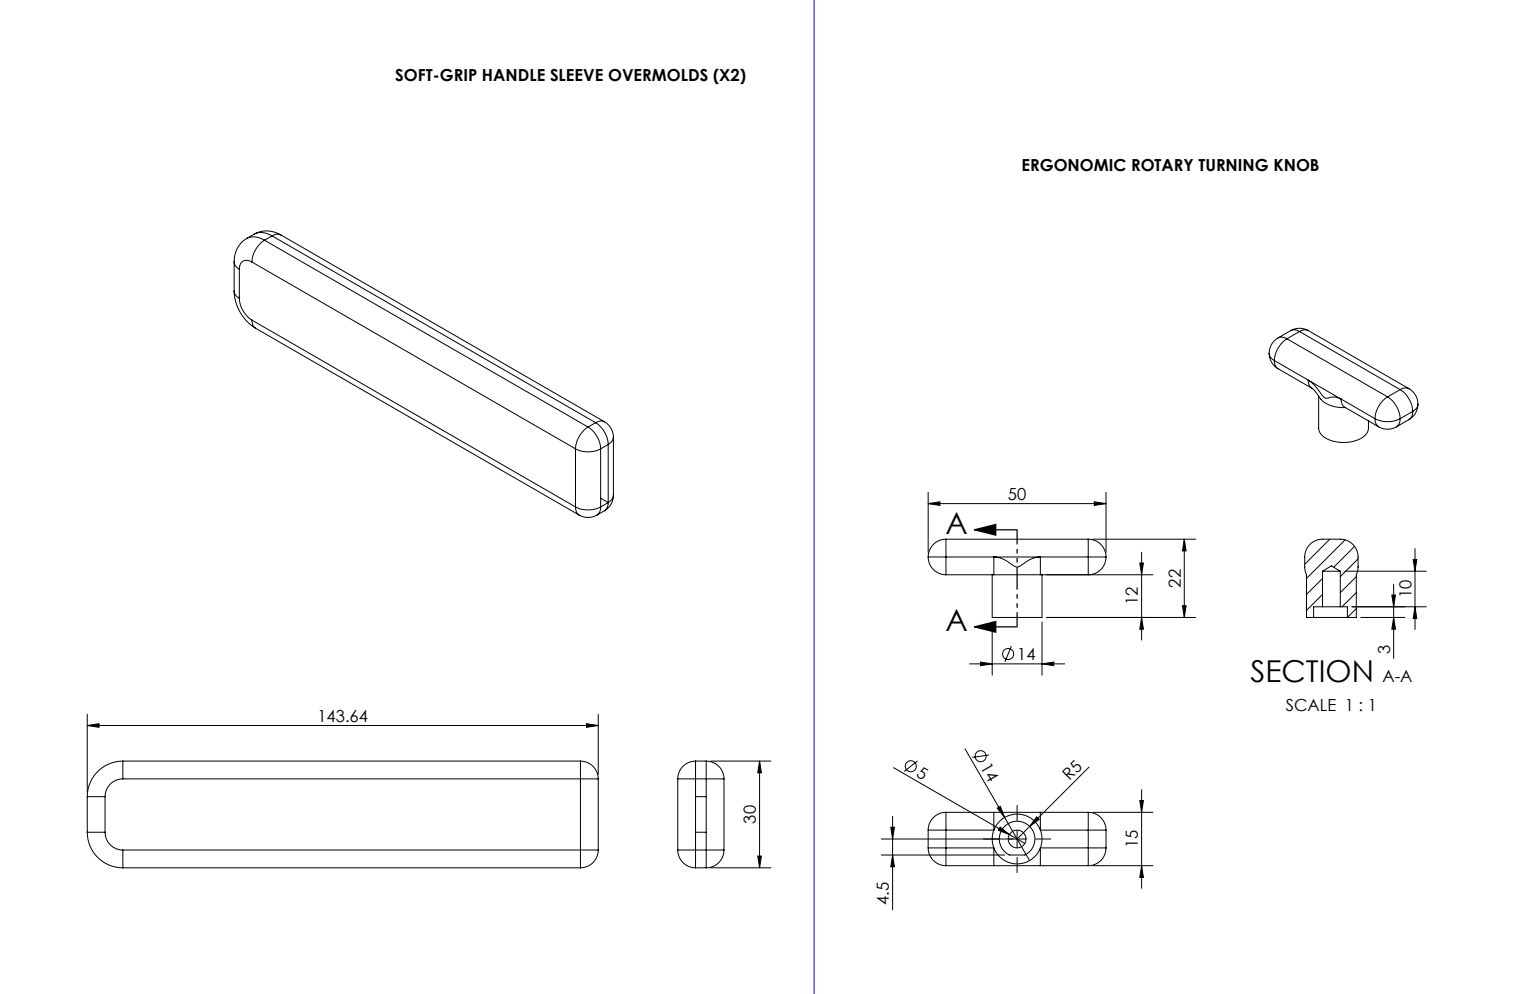
ISO-10303-21;
HEADER;
FILE_DESCRIPTION (('STEP AP214'),
    '1' );
FILE_NAME ('Ergonomic Rotary Turning Knob.step',
    '2026-09-24T10:15:42',
    ( '' ),
    ( '' ),
    'SwSTEP 2.0',
    'SolidWorks 2026',
    '' );
FILE_SCHEMA (( 'AUTOMOTIVE_DESIGN' ));
ENDSEC;

DATA;
#13=CARTESIAN_POINT ( 'NONE',  ( 6.538348415311012296, -7.500000000000000888, -12.00000000000000000 ) ) ;
#17=DIRECTION ( 'NONE',  ( 1.000000000000000000, 0.000000000000000000, 0.000000000000000000 ) ) ;
#23=( BOUNDED_SURFACE ( )  B_SPLINE_SURFACE ( 3, 2, ( 
 ( #9096, #13, #15967 ),
 ( #13391, #10337, #14824 ),
 ( #11773, #4513, #14919 ),
 ( #3147, #1737, #16166 ),
 ( #3050, #14723, #10241 ),
 ( #5830, #6041, #1634 ),
 ( #16367, #7585, #7479 ),
 ( #8709, #13293, #11868 ),
 ( #17403, #308, #4405 ),
 ( #11673, #17708, #11585 ),
 ( #4605, #13483, #14634 ),
 ( #10432, #2857, #16066 ),
 ( #10529, #6137, #4319 ),
 ( #1837, #2958, #14535 ),
 ( #11963, #3250, #7675 ),
 ( #1450, #8805, #1543 ),
 ( #7383, #112, #18081 ),
 ( #4980, #16642, #4896 ),
 ( #1935, #13772, #10817 ),
 ( #3545, #6425, #502 ),
 ( #15014, #6332, #12161 ),
 ( #13684, #7870, #13859 ),
 ( #12251, #7768, #685 ),
 ( #777, #6517, #13581 ),
 ( #598, #3730, #9385 ),
 ( #16464, #9186, #5164 ),
 ( #6228, #10723, #12335 ),
 ( #2209, #3349, #8051 ),
 ( #15212, #12061, #18171 ),
 ( #17895, #2122, #17990 ),
 ( #7963, #5070, #3447 ),
 ( #15113, #9558, #10920 ),
 ( #16558, #16740, #4798 ),
 ( #3639, #11009, #16826 ),
 ( #9474, #15389, #9281 ),
 ( #15296, #6610, #2295 ),
 ( #12433, #18262, #8141 ),
 ( #399, #10633, #2029 ),
 ( #867, #11100, #16916 ),
 ( #5524, #4007, #17020 ),
 ( #5350, #5441, #11374 ),
 ( #2657, #12703, #11287 ),
 ( #17193, #15481, #8406 ),
 ( #6984, #18535, #1038 ) ),
 .UNSPECIFIED., .F., .F., .T. ) 
 B_SPLINE_SURFACE_WITH_KNOTS ( ( 4, 2, 2, 2, 2, 2, 2, 2, 2, 2, 2, 2, 2, 2, 2, 2, 2, 2, 2, 2, 2, 4 ),
 ( 3, 3 ),
 ( 0.007984881688765531685, 0.008880023643941203221, 0.009775165599116873022, 0.01067030755429254282, 0.01156544950946821262, 0.01246059146464388243, 0.01335573341981955396, 0.01425087537499522550, 0.01469844635258306040, 0.01492223184137697785, 0.01514601733017089530, 0.01536980281896481275, 0.01559358830775873020, 0.01581737379655264591, 0.01604115928534656510, 0.01693630124052223490, 0.01783144319569790470, 0.01872658515087357797, 0.01962172710604925124, 0.02051686906122492104, 0.02141201101640059085, 0.02230715297157626065 ),
 ( 0.000000000000000000, 1.000000000000000000 ),
 .UNSPECIFIED. ) 
 GEOMETRIC_REPRESENTATION_ITEM ( )  RATIONAL_B_SPLINE_SURFACE ( (
 ( 1.000000000000000000, 0.7071067811865474617, 1.000000000000000000),
 ( 1.000000000000000000, 0.7141735847353027911, 1.000000000000000000),
 ( 1.000000000000000000, 0.7220150969518837059, 1.000000000000000000),
 ( 1.000000000000000000, 0.7390483610380735868, 1.000000000000000000),
 ( 1.000000000000000000, 0.7482852340371979327, 1.000000000000000000),
 ( 1.000000000000000000, 0.7685052920442676516, 1.000000000000000000),
 ( 1.000000000000000000, 0.7795547470752138830, 1.000000000000000000),
 ( 1.000000000000000000, 0.8031735375541008137, 1.000000000000000000),
 ( 1.000000000000000000, 0.8157770400072400507, 1.000000000000000000),
 ( 1.000000000000000000, 0.8424364036431882807, 1.000000000000000000),
 ( 1.000000000000000000, 0.8565278543580017168, 1.000000000000000000),
 ( 1.000000000000000000, 0.8853337094945018526, 1.000000000000000000),
 ( 1.000000000000000000, 0.9000757013528668526, 1.000000000000000000),
 ( 1.000000000000000000, 0.9285356150544983311, 1.000000000000000000),
 ( 1.000000000000000000, 0.9423225300521810288, 1.000000000000000000),
 ( 1.000000000000000000, 0.9592421851076473605, 1.000000000000000000),
 ( 1.000000000000000000, 0.9642414584271679079, 1.000000000000000000),
 ( 1.000000000000000000, 0.9699277023943830844, 1.000000000000000000),
 ( 1.000000000000000000, 0.9715166551480127755, 1.000000000000000000),
 ( 1.000000000000000000, 0.9737696706145027026, 1.000000000000000000),
 ( 1.000000000000000000, 0.9744508395083844032, 1.000000000000000000),
 ( 1.000000000000000000, 0.9748110790397115366, 1.000000000000000000),
 ( 1.000000000000000000, 0.9744748476087098377, 1.000000000000000000),
 ( 1.000000000000000000, 0.9728601655991807595, 1.000000000000000000),
 ( 1.000000000000000000, 0.9715893508620213614, 1.000000000000000000),
 ( 1.000000000000000000, 0.9682746065025299442, 1.000000000000000000),
 ( 1.000000000000000000, 0.9662330922797159882, 1.000000000000000000),
 ( 1.000000000000000000, 0.9616633680012534047, 1.000000000000000000),
 ( 1.000000000000000000, 0.9591230388079813318, 1.000000000000000000),
 ( 1.000000000000000000, 0.9454866025348970249, 1.000000000000000000),
 ( 1.000000000000000000, 0.9317605398179185094, 1.000000000000000000),
 ( 1.000000000000000000, 0.9032287473899394126, 1.000000000000000000),
 ( 1.000000000000000000, 0.8883390392773794497, 1.000000000000000000),
 ( 1.000000000000000000, 0.8592388025803222584, 1.000000000000000000),
 ( 1.000000000000000000, 0.8450030273492604715, 1.000000000000000000),
 ( 1.000000000000000000, 0.8179255325836626289, 1.000000000000000000),
 ( 1.000000000000000000, 0.8050698650503591569, 1.000000000000000000),
 ( 1.000000000000000000, 0.7808988731588855092, 1.000000000000000000),
 ( 1.000000000000000000, 0.7696290231168715357, 1.000000000000000000),
 ( 1.000000000000000000, 0.7490294503509588031, 1.000000000000000000),
 ( 1.000000000000000000, 0.7396188834547082758, 1.000000000000000000),
 ( 1.000000000000000000, 0.7222670797466549386, 1.000000000000000000),
 ( 1.000000000000000000, 0.7142721232192638103, 1.000000000000000000),
 ( 1.000000000000000000, 0.7071067811865517916, 1.000000000000000000) ) ) 
 REPRESENTATION_ITEM ( '' )  SURFACE ( )  );
#91=B_SPLINE_CURVE_WITH_KNOTS ( 'NONE', 3,
 ( #3030, #15094, #17687, #2012, #6309, #12042, #7847, #10410, #3227, #4588, #16446, #8878, #7562, #11849, #12235, #14704, #7462, #16246, #1615, #18061, #4965, #7658, #8974, #13373, #10511, #16347, #7751, #17876, #9076, #3330, #14902, #9169, #1913, #12143, #13561, #12586, #2450, #12411 ),
 .UNSPECIFIED., .F., .F.,
 ( 4, 2, 2, 2, 2, 2, 2, 2, 2, 2, 2, 2, 2, 2, 2, 2, 2, 2, 4 ),
 ( 0.000000000000000000, 0.0009058109605214417380, 0.001811621921042883476, 0.002717432881564325105, 0.003623243842085765217, 0.004529054802607205762, 0.005434865763128644139, 0.006340676723650081649, 0.006793582203910802572, 0.007246487684171522628, 0.007699393164432242684, 0.008152298644692964474, 0.009058109605214402851, 0.009963920565735844698, 0.01086973152625728828, 0.01177554248677873013, 0.01268135344730017371, 0.01358716440782161729, 0.01449297536834306087 ),
 .UNSPECIFIED. ) ;
#94=CARTESIAN_POINT ( 'NONE',  ( 0.000000000000000000, 0.000000000000000000, -3.000000000000000000 ) ) ;
#97=CARTESIAN_POINT ( 'NONE',  ( -6.538348415311006967, 7.499999999999999112, -17.00000000000000000 ) ) ;
#100=CARTESIAN_POINT ( 'NONE',  ( -6.538348415310934136, -2.500000000000000444, -17.00000000000101252 ) ) ;
#105=EDGE_LOOP ( 'NONE', ( #11918, #3838, #18012, #4953 ) ) ;
#112=CARTESIAN_POINT ( 'NONE',  ( 1.213280723413316275, -7.500000000000199840, -13.07603167631435603 ) ) ;
#115=DIRECTION ( 'NONE',  ( 0.000000000000000000, 0.000000000000000000, 1.000000000000000000 ) ) ;
#128=ORIENTED_EDGE ( 'NONE', *, *, #3767, .F. ) ;
#158=ORIENTED_EDGE ( 'NONE', *, *, #3779, .F. ) ;
#183=ORIENTED_EDGE ( 'NONE', *, *, #15931, .F. ) ;
#186=DIRECTION ( 'NONE',  ( 0.000000000000000000, 0.000000000000000000, -1.000000000000000000 ) ) ;
#189=DIRECTION ( 'NONE',  ( -1.000000000000000000, -8.673617379884033500E-16, 0.000000000000000000 ) ) ;
#194=CARTESIAN_POINT ( 'NONE',  ( 25.00000000000000000, 7.499999999999999112, -16.99999999999999645 ) ) ;
#197=ORIENTED_EDGE ( 'NONE', *, *, #8046, .T. ) ;
#226=AXIS2_PLACEMENT_3D ( 'NONE', #9917, #9039, #13430 ) ;
#229=CARTESIAN_POINT ( 'NONE',  ( 0.000000000000000000, 0.000000000000000000, -12.00000000000000000 ) ) ;
#230=EDGE_LOOP ( 'NONE', ( #7603, #4176, #7702, #11957 ) ) ;
#232=ORIENTED_EDGE ( 'NONE', *, *, #17218, .F. ) ;
#253=ORIENTED_EDGE ( 'NONE', *, *, #15488, .F. ) ;
#270=CARTESIAN_POINT ( 'NONE',  ( 2.179449471770337432, -4.500000000000000000, -3.000000000000000000 ) ) ;
#289=DIRECTION ( 'NONE',  ( -0.000000000000000000, -0.000000000000000000, 1.000000000000000000 ) ) ;
#290=CARTESIAN_POINT ( 'NONE',  ( -5.935721797379079234, 7.499999999999999112, -16.97606798286715701 ) ) ;
#298=AXIS2_PLACEMENT_3D ( 'NONE', #7660, #11852, #11947 ) ;
#308=CARTESIAN_POINT ( 'NONE',  ( 5.084818453916919445, -7.499999999999999112, -13.03762002034291534 ) ) ;
#316=DIRECTION ( 'NONE',  ( -1.000000000000000000, 1.734723475976806848E-16, 0.000000000000000000 ) ) ;
#322=VERTEX_POINT ( 'NONE', #3941 ) ;
#370=ORIENTED_EDGE ( 'NONE', *, *, #6465, .T. ) ;
#376=DIRECTION ( 'NONE',  ( 0.000000000000000000, -0.000000000000000000, 1.000000000000000000 ) ) ;
#393=ORIENTED_EDGE ( 'NONE', *, *, #1315, .T. ) ;
#394=CARTESIAN_POINT ( 'NONE',  ( 20.00000000000000000, -2.500000000000000444, -17.00000000000000000 ) ) ;
#399=CARTESIAN_POINT ( 'NONE',  ( -6.009712068683241704, -3.596569907853852666, -12.00000000129638345 ) ) ;
#412=DIRECTION ( 'NONE',  ( 1.000000000000000000, -0.000000000000000000, -0.000000000000000000 ) ) ;
#435=SURFACE_STYLE_USAGE ( .BOTH. , #6368 ) ;
#437=DIRECTION ( 'NONE',  ( -0.000000000000000000, -1.000000000000000000, -0.000000000000000000 ) ) ;
#465=DIRECTION ( 'NONE',  ( -1.000000000000000000, -0.000000000000000000, -0.000000000000000000 ) ) ;
#467=DIRECTION ( 'NONE',  ( 1.000000000000000000, 0.000000000000000000, -0.000000000000000000 ) ) ;
#481=ORIENTED_EDGE ( 'NONE', *, *, #8485, .T. ) ;
#483=FACE_OUTER_BOUND ( 'NONE', #969, .T. ) ;
#502=CARTESIAN_POINT ( 'NONE',  ( 0.1927609796801927344, -7.500000000000000888, -14.19253746125320781 ) ) ;
#528=AXIS2_PLACEMENT_3D ( 'NONE', #16332, #14594, #1513 ) ;
#540=( NAMED_UNIT ( * ) SI_UNIT ( $, .STERADIAN. ) SOLID_ANGLE_UNIT ( ) );
#558=DIRECTION ( 'NONE',  ( 0.000000000000000000, -0.000000000000000000, 1.000000000000000000 ) ) ;
#569=AXIS2_PLACEMENT_3D ( 'NONE', #9771, #3860, #988 ) ;
#582=CARTESIAN_POINT ( 'NONE',  ( -20.00000000000000000, 2.499999999999998668, -16.99999999999999645 ) ) ;
#583=CARTESIAN_POINT ( 'NONE',  ( -5.052632128771760378, 7.499999999999999112, -16.81774875490144083 ) ) ;
#598=CARTESIAN_POINT ( 'NONE',  ( -0.9371186270710654131, -6.939831204821797606, -11.99999999628260916 ) ) ;
#605=CIRCLE ( 'NONE', #298, 5.000000000000000888 ) ;
#622=VERTEX_POINT ( 'NONE', #3146 ) ;
#643=CARTESIAN_POINT ( 'NONE',  ( -20.00000000000000000, 2.499999999999998668, -16.99999999999999645 ) ) ;
#659=DIRECTION ( 'NONE',  ( 0.000000000000000000, 1.000000000000000000, 0.000000000000000000 ) ) ;
#671=CARTESIAN_POINT ( 'NONE',  ( -4.545271119322114473, 5.336083332029744497, -11.99999999554324681 ) ) ;
#684=PRODUCT ( 'Ergonomic Rotary Turning Knob', 'Ergonomic Rotary Turning Knob', '', ( #12370 ) ) ;
#685=CARTESIAN_POINT ( 'NONE',  ( -0.1127451301830492136, -7.500000000000000888, -14.18240585847551571 ) ) ;
#724=FACE_BOUND ( 'NONE', #4955, .T. ) ;
#744=EDGE_CURVE ( 'NONE', #7194, #11848, #2712, .T. ) ;
#748=VERTEX_POINT ( 'NONE', #3729 ) ;
#759=CARTESIAN_POINT ( 'NONE',  ( -5.641944871949442941, 4.153144983957288261, -12.00000000256090260 ) ) ;
#766=AXIS2_PLACEMENT_3D ( 'NONE', #12959, #3987, #2814 ) ;
#770=ORIENTED_EDGE ( 'NONE', *, *, #1831, .T. ) ;
#777=CARTESIAN_POINT ( 'NONE',  ( -0.7340363079797833645, -6.964562493341727389, -12.00000000352072504 ) ) ;
#807=LINE ( 'NONE', #18293, #15132 ) ;
#823=CARTESIAN_POINT ( 'NONE',  ( 4.195027931520234787, -7.500000000000001776, -16.53644619669688254 ) ) ;
#827=FACE_OUTER_BOUND ( 'NONE', #6255, .T. ) ;
#828=DIRECTION ( 'NONE',  ( -1.000000000000000000, 0.000000000000000000, 0.000000000000000000 ) ) ;
#833=CARTESIAN_POINT ( 'NONE',  ( 25.00000000000000000, 7.499999999999999112, -16.99999999999999645 ) ) ;
#837=ORIENTED_EDGE ( 'NONE', *, *, #10654, .T. ) ;
#852=CARTESIAN_POINT ( 'NONE',  ( -6.344274892086297690, 2.961199469785570138, -11.99999999981461585 ) ) ;
#854=AXIS2_PLACEMENT_3D ( 'NONE', #15349, #9347, #10785 ) ;
#867=CARTESIAN_POINT ( 'NONE',  ( -6.108979705494616219, -3.422227477007855789, -11.99999999936559902 ) ) ;
#876=CARTESIAN_POINT ( 'NONE',  ( 20.00000000000000000, 2.499999999999998668, -17.00000000000000000 ) ) ;
#915=CARTESIAN_POINT ( 'NONE',  ( -4.160991745704744282, -7.500000000000002665, -16.52287405655582475 ) ) ;
#938=CARTESIAN_POINT ( 'NONE',  ( 6.453131650770538741, 2.715944631655133001, -12.00000000019078428 ) ) ;
#968=DIRECTION ( 'NONE',  ( 1.000000000000000000, 0.000000000000000000, 0.000000000000000000 ) ) ;
#969=EDGE_LOOP ( 'NONE', ( #5849, #9714, #10891, #1040, #8292, #7403 ) ) ;
#981=AXIS2_PLACEMENT_3D ( 'NONE', #15850, #2740, #2928 ) ;
#988=DIRECTION ( 'NONE',  ( 1.000000000000000000, 0.000000000000000000, -0.000000000000000000 ) ) ;
#1026=ADVANCED_FACE ( 'NONE', ( #14896 ), #12138, .T. ) ;
#1027=DIRECTION ( 'NONE',  ( -1.000000000000000000, 0.000000000000000000, 0.000000000000000000 ) ) ;
#1038=CARTESIAN_POINT ( 'NONE',  ( -6.538348415310826667, -7.500000000000000888, -17.00000000000000000 ) ) ;
#1039=LINE ( 'NONE', #4919, #11473 ) ;
#1040=ORIENTED_EDGE ( 'NONE', *, *, #8176, .F. ) ;
#1065=CIRCLE ( 'NONE', #13280, 7.000000000000000000 ) ;
#1096=DIRECTION ( 'NONE',  ( 0.000000000000000000, 0.000000000000000000, -1.000000000000000000 ) ) ;
#1116=CARTESIAN_POINT ( 'NONE',  ( 5.926008024970927934, 7.499999999999999112, -16.97528233579637558 ) ) ;
#1123=AXIS2_PLACEMENT_3D ( 'NONE', #6884, #14137, #3641 ) ;
#1149=CARTESIAN_POINT ( 'NONE',  ( 7.000000000000000000, 0.000000000000000000, -12.00000000000000000 ) ) ;
#1161=ORIENTED_EDGE ( 'NONE', *, *, #10654, .F. ) ;
#1179=CARTESIAN_POINT ( 'NONE',  ( -20.00000000000000000, -7.500000000000000888, -12.00000000000000000 ) ) ;
#1187=VERTEX_POINT ( 'NONE', #2444 ) ;
#1195=CARTESIAN_POINT ( 'NONE',  ( 20.00000000000000000, 2.499999999999998668, -16.99999999999999645 ) ) ;
#1209=CYLINDRICAL_SURFACE ( 'NONE', #766, 5.000000000000000888 ) ;
#1211=CARTESIAN_POINT ( 'NONE',  ( 1.517261107235507778, 6.836011689345040665, -11.99999999467225997 ) ) ;
#1222=ORIENTED_EDGE ( 'NONE', *, *, #14362, .F. ) ;
#1229=ADVANCED_FACE ( 'NONE', ( #14392 ), #17355, .T. ) ;
#1268=CARTESIAN_POINT ( 'NONE',  ( 20.00000000000000000, -7.500000000000000888, -17.00000000000000000 ) ) ;
#1280=CYLINDRICAL_SURFACE ( 'NONE', #14175, 5.000000000000000000 ) ;
#1296=ORIENTED_EDGE ( 'NONE', *, *, #18671, .F. ) ;
#1299=CARTESIAN_POINT ( 'NONE',  ( 20.00000000000000000, 2.499999999999998668, -16.99999999999999645 ) ) ;
#1305=CARTESIAN_POINT ( 'NONE',  ( 1.870513085853429791, 6.747912118474282295, -12.00000000532774003 ) ) ;
#1315=EDGE_CURVE ( 'NONE', #12766, #16531, #8955, .T. ) ;
#1329=DIRECTION ( 'NONE',  ( 0.000000000000000000, -0.000000000000000000, 1.000000000000000000 ) ) ;
#1332=DIRECTION ( 'NONE',  ( 0.000000000000000000, 0.000000000000000000, 1.000000000000000000 ) ) ;
#1350=CARTESIAN_POINT ( 'NONE',  ( 0.000000000000000000, 0.000000000000000000, -3.000000000000000000 ) ) ;
#1357=ORIENTED_EDGE ( 'NONE', *, *, #7230, .T. ) ;
#1366=VECTOR ( 'NONE', #18178, 1000.000000000000000 ) ;
#1379=DIRECTION ( 'NONE',  ( 0.000000000000000000, 0.000000000000000000, 1.000000000000000000 ) ) ;
#1392=ORIENTED_EDGE ( 'NONE', *, *, #8942, .F. ) ;
#1450=CARTESIAN_POINT ( 'NONE',  ( 2.048748540252052663, -6.701137625570377843, -11.99999999225501668 ) ) ;
#1462=CARTESIAN_POINT ( 'NONE',  ( -7.000000000000000000, 8.572527594031473190E-16, 0.000000000000000000 ) ) ;
#1466=ORIENTED_EDGE ( 'NONE', *, *, #7516, .T. ) ;
#1468=ORIENTED_EDGE ( 'NONE', *, *, #9424, .T. ) ;
#1499=DIRECTION ( 'NONE',  ( 0.000000000000000000, 0.000000000000000000, 1.000000000000000000 ) ) ;
#1513=DIRECTION ( 'NONE',  ( 0.000000000000000000, 0.000000000000000000, -1.000000000000000000 ) ) ;
#1514=AXIS2_PLACEMENT_3D ( 'NONE', #8574, #14398, #8664 ) ;
#1543=CARTESIAN_POINT ( 'NONE',  ( 0.7622588538374807099, -7.500000000000000888, -14.39637362139749932 ) ) ;
#1576=( LENGTH_UNIT ( ) NAMED_UNIT ( * ) SI_UNIT ( .MILLI., .METRE. ) );
#1615=CARTESIAN_POINT ( 'NONE',  ( -0.1940040276537092212, 7.499999999999998224, -14.18536928022391663 ) ) ;
#1627=CIRCLE ( 'NONE', #10178, 5.000000000000000888 ) ;
#1634=CARTESIAN_POINT ( 'NONE',  ( 4.479409541426081276, -7.500000000000000888, -16.64412940056557488 ) ) ;
#1637=ADVANCED_FACE ( 'NONE', ( #2769 ), #14443, .F. ) ;
#1641=COLOUR_RGB ( '', 0.66274510, 0.83137255, 0.94901961) ;
#1646=CARTESIAN_POINT ( 'NONE',  ( 0.000000000000000000, 0.000000000000000000, -3.000000000000000000 ) ) ;
#1669=DIRECTION ( 'NONE',  ( 0.000000000000000000, 0.000000000000000000, -1.000000000000000000 ) ) ;
#1689=DIRECTION ( 'NONE',  ( -0.000000000000000000, -1.000000000000000000, -0.000000000000000000 ) ) ;
#1698=CARTESIAN_POINT ( 'NONE',  ( 25.00000000000000000, -2.500000000000000444, -17.00000000000000000 ) ) ;
#1716=CIRCLE ( 'NONE', #6298, 5.000000000000000888 ) ;
#1736=UNCERTAINTY_MEASURE_WITH_UNIT (LENGTH_MEASURE( 1.000000000000000082E-05 ), #1576, 'distance_accuracy_value', 'NONE');
#1737=CARTESIAN_POINT ( 'NONE',  ( 6.265543861956754057, -7.499999999999872990, -12.41474642440651621 ) ) ;
#1772=( NAMED_UNIT ( * ) PLANE_ANGLE_UNIT ( ) SI_UNIT ( $, .RADIAN. ) );
#1773=CARTESIAN_POINT ( 'NONE',  ( 0.000000000000000000, 0.000000000000000000, 0.000000000000000000 ) ) ;
#1785=ORIENTED_EDGE ( 'NONE', *, *, #12342, .T. ) ;
#1807=VERTEX_POINT ( 'NONE', #17106 ) ;
#1821=DIRECTION ( 'NONE',  ( -1.000000000000000000, -0.000000000000000000, -0.000000000000000000 ) ) ;
#1829=CARTESIAN_POINT ( 'NONE',  ( -25.00000000000000000, 2.499999999999998668, -12.00000000000000000 ) ) ;
#1831=EDGE_CURVE ( 'NONE', #16711, #12401, #4496, .T. ) ;
#1832=EDGE_CURVE ( 'NONE', #16531, #4154, #12338, .T. ) ;
#1837=CARTESIAN_POINT ( 'NONE',  ( 3.431439422793015392, -6.119758975832682246, -11.99999999209394907 ) ) ;
#1844=ADVANCED_FACE ( 'NONE', ( #14055 ), #5167, .T. ) ;
#1856=ORIENTED_EDGE ( 'NONE', *, *, #10608, .T. ) ;
#1894=DIRECTION ( 'NONE',  ( -0.000000000000000000, -1.000000000000000000, 0.000000000000000000 ) ) ;
#1913=CARTESIAN_POINT ( 'NONE',  ( 4.447775431366602916, 7.499999999999999112, -16.63307795419225599 ) ) ;
#1923=( BOUNDED_SURFACE ( )  B_SPLINE_SURFACE ( 3, 2, ( 
 ( #16150, #10412, #97 ),
 ( #11754, #16248, #3130 ),
 ( #14806, #7566, #290 ),
 ( #852, #10803, #14034 ),
 ( #8216, #5147, #583 ),
 ( #6311, #8126, #12146 ),
 ( #3530, #6408, #15461 ),
 ( #16725, #17976, #4880 ),
 ( #759, #10708, #6688 ),
 ( #7950, #3625, #16544 ),
 ( #9461, #3806, #3429 ),
 ( #671, #15283, #9266 ),
 ( #8035, #2276, #7850 ),
 ( #15370, #18249, #15096 ),
 ( #18332, #13936, #2014 ),
 ( #11085, #2194, #12502 ),
 ( #13670, #5241, #18153 ),
 ( #10904, #13843, #2369 ),
 ( #12239, #16900, #9634 ),
 ( #18063, #4968, #13756 ),
 ( #16629, #9365, #15197 ),
 ( #2110, #6500, #16811 ),
 ( #12323, #5055, #6592 ),
 ( #12416, #10995, #3715 ),
 ( #9542, #8389, #16998 ),
 ( #18419, #10101, #17362 ),
 ( #1211, #3903, #5691 ),
 ( #1305, #6967, #2728 ),
 ( #8573, #2639, #7149 ),
 ( #12867, #14313, #9907 ),
 ( #12778, #10002, #7056 ),
 ( #5423, #17087, #14220 ),
 ( #4278, #6779, #15737 ),
 ( #18694, #18515, #4188 ),
 ( #11543, #14397, #8483 ),
 ( #2451, #5596, #11447 ),
 ( #12686, #18604, #15834 ),
 ( #2539, #12962, #17265 ),
 ( #6865, #15927, #8302 ),
 ( #11270, #18793, #3992 ),
 ( #8662, #15637, #2816 ),
 ( #938, #12589, #1116 ),
 ( #5332, #11176, #5507 ),
 ( #9727, #15554, #14116 ) ),
 .UNSPECIFIED., .F., .F., .T. ) 
 B_SPLINE_SURFACE_WITH_KNOTS ( ( 4, 2, 2, 2, 2, 2, 2, 2, 2, 2, 2, 2, 2, 2, 2, 2, 2, 2, 2, 2, 2, 4 ),
 ( 3, 3 ),
 ( 0.007984881688765545563, 0.008880023643941227507, 0.009775165599116911186, 0.01067030755429259313, 0.01156544950946827507, 0.01246059146464395875, 0.01335573341981964070, 0.01425087537499532264, 0.01469844635258316448, 0.01492223184137708540, 0.01514601733017100632, 0.01536980281896492724, 0.01559358830775884816, 0.01581737379655277081, 0.01604115928534669000, 0.01693630124052237021, 0.01783144319569805042, 0.01872658515087373410, 0.01962172710604941778, 0.02051686906122510146, 0.02141201101640078513, 0.02230715297157646534 ),
 ( 0.000000000000000000, 1.000000000000000000 ),
 .UNSPECIFIED. ) 
 GEOMETRIC_REPRESENTATION_ITEM ( )  RATIONAL_B_SPLINE_SURFACE ( (
 ( 1.000000000000000000, 0.7071067811865475727, 1.000000000000000000),
 ( 1.000000000000000000, 0.7141735847352902455, 1.000000000000000000),
 ( 1.000000000000000000, 0.7220150969519002482, 1.000000000000000000),
 ( 1.000000000000000000, 0.7390483610380570445, 1.000000000000000000),
 ( 1.000000000000000000, 0.7482852340372653233, 1.000000000000000000),
 ( 1.000000000000000000, 0.7685052920442022595, 1.000000000000000000),
 ( 1.000000000000000000, 0.7795547470751481578, 1.000000000000000000),
 ( 1.000000000000000000, 0.8031735375541687594, 1.000000000000000000),
 ( 1.000000000000000000, 0.8157770400072592576, 1.000000000000000000),
 ( 1.000000000000000000, 0.8424364036431745140, 1.000000000000000000),
 ( 1.000000000000000000, 0.8565278543580376880, 1.000000000000000000),
 ( 1.000000000000000000, 0.8853337094944713215, 1.000000000000000000),
 ( 1.000000000000000000, 0.9000757013528374317, 1.000000000000000000),
 ( 1.000000000000000000, 0.9285356150545359677, 1.000000000000000000),
 ( 1.000000000000000000, 0.9423225300521840264, 1.000000000000000000),
 ( 1.000000000000000000, 0.9592421851076505801, 1.000000000000000000),
 ( 1.000000000000000000, 0.9642414584271785660, 1.000000000000000000),
 ( 1.000000000000000000, 0.9699277023943811971, 1.000000000000000000),
 ( 1.000000000000000000, 0.9715166551480145518, 1.000000000000000000),
 ( 1.000000000000000000, 0.9737696706145044789, 1.000000000000000000),
 ( 1.000000000000000000, 0.9744508395083761876, 1.000000000000000000),
 ( 1.000000000000000000, 0.9748110790397204184, 1.000000000000000000),
 ( 1.000000000000000000, 0.9744748476087129463, 1.000000000000000000),
 ( 1.000000000000000000, 0.9728601655991754305, 1.000000000000000000),
 ( 1.000000000000000000, 0.9715893508620192520, 1.000000000000000000),
 ( 1.000000000000000000, 0.9682746065025277238, 1.000000000000000000),
 ( 1.000000000000000000, 0.9662330922797167654, 1.000000000000000000),
 ( 1.000000000000000000, 0.9616633680012457441, 1.000000000000000000),
 ( 1.000000000000000000, 0.9591230388079776681, 1.000000000000000000),
 ( 1.000000000000000000, 0.9454866025348932501, 1.000000000000000000),
 ( 1.000000000000000000, 0.9317605398179132914, 1.000000000000000000),
 ( 1.000000000000000000, 0.9032287473899339725, 1.000000000000000000),
 ( 1.000000000000000000, 0.8883390392773735655, 1.000000000000000000),
 ( 1.000000000000000000, 0.8592388025803160412, 1.000000000000000000),
 ( 1.000000000000000000, 0.8450030273492536992, 1.000000000000000000),
 ( 1.000000000000000000, 0.8179255325836554125, 1.000000000000000000),
 ( 1.000000000000000000, 0.8050698650503534948, 1.000000000000000000),
 ( 1.000000000000000000, 0.7808988731588796250, 1.000000000000000000),
 ( 1.000000000000000000, 0.7696290231168499973, 1.000000000000000000),
 ( 1.000000000000000000, 0.7490294503509707935, 1.000000000000000000),
 ( 1.000000000000000000, 0.7396188834547036128, 1.000000000000000000),
 ( 1.000000000000000000, 0.7222670797466500536, 1.000000000000000000),
 ( 1.000000000000000000, 0.7142721232192589254, 1.000000000000000000),
 ( 1.000000000000000000, 0.7071067811865474617, 1.000000000000000000) ) ) 
 REPRESENTATION_ITEM ( '' )  SURFACE ( )  );
#1928=CARTESIAN_POINT ( 'NONE',  ( 25.00000000000000000, 7.499999999999999112, -17.00000000000000000 ) ) ;
#1929=ORIENTED_EDGE ( 'NONE', *, *, #4337, .F. ) ;
#1930=DIRECTION ( 'NONE',  ( 0.000000000000000000, 1.734723475976806700E-15, -1.000000000000000000 ) ) ;
#1932=CIRCLE ( 'NONE', #10475, 5.000000000000000888 ) ;
#1935=CARTESIAN_POINT ( 'NONE',  ( 0.9490252293518500748, -6.938433416811018439, -12.00000000290481594 ) ) ;
#1939=DIRECTION ( 'NONE',  ( 1.000000000000000000, 0.000000000000000000, 0.000000000000000000 ) ) ;
#1955=ADVANCED_FACE ( 'NONE', ( #7366, #6988 ), #13178, .T. ) ;
#1959=VECTOR ( 'NONE', #7017, 1000.000000000000000 ) ;
#2012=CARTESIAN_POINT ( 'NONE',  ( -5.342326914280422834, 7.500000000000000000, -16.88455910646440827 ) ) ;
#2014=CARTESIAN_POINT ( 'NONE',  ( -1.149093537842120316, 7.499999999999999112, -14.62468756229416300 ) ) ;
#2015=CARTESIAN_POINT ( 'NONE',  ( 0.000000000000000000, 0.000000000000000000, -14.50215154756889824 ) ) ;
#2017=SURFACE_STYLE_USAGE ( .BOTH. , #16547 ) ;
#2026=ORIENTED_EDGE ( 'NONE', *, *, #9182, .F. ) ;
#2029=CARTESIAN_POINT ( 'NONE',  ( -4.162578369387166077, -7.500000000000000888, -16.52352554129683426 ) ) ;
#2030=AXIS2_PLACEMENT_3D ( 'NONE', #15716, #11248, #17249 ) ;
#2038=DIRECTION ( 'NONE',  ( -1.000000000000000000, 0.000000000000000000, 0.000000000000000000 ) ) ;
#2048=EDGE_CURVE ( 'NONE', #17649, #12162, #91, .T. ) ;
#2058=CARTESIAN_POINT ( 'NONE',  ( 25.00000000000000000, 2.499999999999997780, -17.00000000000000000 ) ) ;
#2066=PRESENTATION_STYLE_ASSIGNMENT (( #435 ) ) ;
#2086=CARTESIAN_POINT ( 'NONE',  ( -6.538348415311014072, -7.500000000000000888, -16.99999999999999645 ) ) ;
#2088=CARTESIAN_POINT ( 'NONE',  ( -6.538348415311014072, 7.499999999999999112, -16.99999999999999645 ) ) ;
#2093=CARTESIAN_POINT ( 'NONE',  ( 20.00000000000000000, -2.500000000000000444, -17.00000000000000000 ) ) ;
#2110=CARTESIAN_POINT ( 'NONE',  ( 0.09864563712547316787, 7.002566078024234919, -11.99999999788117044 ) ) ;
#2111=FACE_OUTER_BOUND ( 'NONE', #10163, .T. ) ;
#2113=( LENGTH_UNIT ( ) NAMED_UNIT ( * ) SI_UNIT ( .MILLI., .METRE. ) );
#2122=CARTESIAN_POINT ( 'NONE',  ( -2.061733300930191692, -7.500000000000532019, -13.14107379030518530 ) ) ;
#2123=ORIENTED_EDGE ( 'NONE', *, *, #17662, .T. ) ;
#2131=CIRCLE ( 'NONE', #14618, 7.000000000000000000 ) ;
#2154=ADVANCED_FACE ( 'NONE', ( #4081 ), #1209, .T. ) ;
#2155=( NAMED_UNIT ( * ) PLANE_ANGLE_UNIT ( ) SI_UNIT ( $, .RADIAN. ) );
#2161=DIRECTION ( 'NONE',  ( 0.000000000000000000, 0.000000000000000000, -1.000000000000000000 ) ) ;
#2174=DIRECTION ( 'NONE',  ( -0.000000000000000000, 1.000000000000000000, -0.000000000000000000 ) ) ;
#2194=CARTESIAN_POINT ( 'NONE',  ( -1.461502493107204925, 7.500000000000000888, -13.09494173305782994 ) ) ;
#2209=CARTESIAN_POINT ( 'NONE',  ( -1.870513085853194424, -6.747912118474371113, -12.00000000532778266 ) ) ;
#2220=CARTESIAN_POINT ( 'NONE',  ( 2.179449471770337432, -4.500000000000000000, -3.000000000000000000 ) ) ;
#2232=DIRECTION ( 'NONE',  ( -0.000000000000000000, -0.000000000000000000, 1.000000000000000000 ) ) ;
#2246=ADVANCED_FACE ( 'NONE', ( #13535 ), #7726, .T. ) ;
#2253=CARTESIAN_POINT ( 'NONE',  ( -1.088636994872529185, -7.500000000000003553, -14.58255216580684888 ) ) ;
#2276=CARTESIAN_POINT ( 'NONE',  ( -3.329573251201238815, 7.500000000000000888, -13.21489263293670113 ) ) ;
#2289=AXIS2_PLACEMENT_3D ( 'NONE', #8684, #8591, #14413 ) ;
#2292=EDGE_LOOP ( 'NONE', ( #17599, #5760, #5139, #1468 ) ) ;
#2295=CARTESIAN_POINT ( 'NONE',  ( -3.338474662713250662, -7.500000000000000888, -16.12819240262148668 ) ) ;
#2297=DIRECTION ( 'NONE',  ( 0.000000000000000000, 0.000000000000000000, 1.000000000000000000 ) ) ;
#2325=EDGE_CURVE ( 'NONE', #5848, #17372, #4463, .T. ) ;
#2346=SPHERICAL_SURFACE ( 'NONE', #2596, 5.000000000000000000 ) ;
#2369=CARTESIAN_POINT ( 'NONE',  ( -0.4158217634471630397, 7.499999999999999112, -14.24727159067854387 ) ) ;
#2377=EDGE_CURVE ( 'NONE', #3494, #13344, #6463, .T. ) ;
#2389=DIRECTION ( 'NONE',  ( -0.000000000000000000, -0.000000000000000000, 1.000000000000000000 ) ) ;
#2392=ADVANCED_FACE ( 'NONE', ( #6383 ), #8279, .T. ) ;
#2418=FACE_OUTER_BOUND ( 'NONE', #2292, .T. ) ;
#2421=AXIS2_PLACEMENT_3D ( 'NONE', #9557, #5349, #6879 ) ;
#2431=CARTESIAN_POINT ( 'NONE',  ( -2.563381608035275594, -7.500000000000003553, -15.65171369207284791 ) ) ;
#2432=DIRECTION ( 'NONE',  ( 1.000000000000000000, 0.000000000000000000, 0.000000000000000000 ) ) ;
#2441=ADVANCED_FACE ( 'NONE', ( #15615 ), #1280, .F. ) ;
#2444=CARTESIAN_POINT ( 'NONE',  ( -5.000000000000000000, 6.123233995736766282E-16, -3.000000000000000000 ) ) ;
#2450=CARTESIAN_POINT ( 'NONE',  ( 6.231098469233193882, 7.500000000000000000, -17.00000000000000000 ) ) ;
#2451=CARTESIAN_POINT ( 'NONE',  ( 5.616333669597326050, 4.188188789804502044, -12.00000000261158917 ) ) ;
#2455=CARTESIAN_POINT ( 'NONE',  ( 0.000000000000000000, 0.000000000000000000, -12.00000000000000000 ) ) ;
#2463=EDGE_CURVE ( 'NONE', #9741, #9678, #8379, .T. ) ;
#2465=EDGE_CURVE ( 'NONE', #322, #12162, #9670, .T. ) ;
#2515=DIRECTION ( 'NONE',  ( 0.000000000000000000, 0.000000000000000000, -1.000000000000000000 ) ) ;
#2519=DIRECTION ( 'NONE',  ( -1.000000000000000000, 0.000000000000000000, 0.000000000000000000 ) ) ;
#2525=ORIENTED_EDGE ( 'NONE', *, *, #9512, .F. ) ;
#2527=ORIENTED_EDGE ( 'NONE', *, *, #744, .F. ) ;
#2539=CARTESIAN_POINT ( 'NONE',  ( 6.009712068683786157, 3.596569907853440551, -12.00000000129651312 ) ) ;
#2589=CARTESIAN_POINT ( 'NONE',  ( 5.000000000000000000, 0.000000000000000000, -3.000000000000000000 ) ) ;
#2596=AXIS2_PLACEMENT_3D ( 'NONE', #13911, #2432, #17247 ) ;
#2599=DIRECTION ( 'NONE',  ( -0.000000000000000000, -0.000000000000000000, 1.000000000000000000 ) ) ;
#2611=MECHANICAL_DESIGN_GEOMETRIC_PRESENTATION_REPRESENTATION('',(#10889),#16049);
#2616=FACE_OUTER_BOUND ( 'NONE', #12084, .T. ) ;
#2639=CARTESIAN_POINT ( 'NONE',  ( 1.454043889487796948, 7.500000000000062172, -13.09460583645960696 ) ) ;
#2657=CARTESIAN_POINT ( 'NONE',  ( -6.453131650770636440, -2.715944631655204056, -12.00000000019080382 ) ) ;
#2672=DIRECTION ( 'NONE',  ( -0.000000000000000000, -0.000000000000000000, 1.000000000000000000 ) ) ;
#2691=CARTESIAN_POINT ( 'NONE',  ( 2.500000000000000000, 0.000000000000000000, -3.000000000000000000 ) ) ;
#2692=ORIENTED_EDGE ( 'NONE', *, *, #10424, .T. ) ;
#2712=CIRCLE ( 'NONE', #2421, 5.000000000000000000 ) ;
#2713=AXIS2_PLACEMENT_3D ( 'NONE', #16698, #1894, #5128 ) ;
#2728=CARTESIAN_POINT ( 'NONE',  ( 0.6925461861255360896, 7.499999999999999112, -14.36265820198533483 ) ) ;
#2740=DIRECTION ( 'NONE',  ( -1.000000000000000000, -0.000000000000000000, -0.000000000000000000 ) ) ;
#2758=ORIENTED_EDGE ( 'NONE', *, *, #11526, .F. ) ;
#2760=CARTESIAN_POINT ( 'NONE',  ( -20.00000000000000000, -7.500000000000000888, -16.99999999999999645 ) ) ;
#2769=FACE_OUTER_BOUND ( 'NONE', #11793, .T. ) ;
#2794=DIRECTION ( 'NONE',  ( 0.000000000000000000, 0.000000000000000000, 1.000000000000000000 ) ) ;
#2809=ORIENTED_EDGE ( 'NONE', *, *, #17661, .F. ) ;
#2814=DIRECTION ( 'NONE',  ( 0.000000000000000000, 0.000000000000000000, 1.000000000000000000 ) ) ;
#2816=CARTESIAN_POINT ( 'NONE',  ( 5.324905852943008000, 7.499999999999999112, -16.88120503408576312 ) ) ;
#2857=CARTESIAN_POINT ( 'NONE',  ( 3.669726844813488764, -7.499999999999743316, -13.21471411064825396 ) ) ;
#2861=DIRECTION ( 'NONE',  ( -0.000000000000000000, -0.000000000000000000, 1.000000000000000000 ) ) ;
#2871=CARTESIAN_POINT ( 'NONE',  ( 0.000000000000000000, -2.500000000000000444, -22.00000000000000000 ) ) ;
#2873=AXIS2_PLACEMENT_3D ( 'NONE', #14246, #14422, #1332 ) ;
#2883=LINE ( 'NONE', #13129, #9817 ) ;
#2928=DIRECTION ( 'NONE',  ( 0.000000000000000000, 0.000000000000000000, 1.000000000000000000 ) ) ;
#2937=ORIENTED_EDGE ( 'NONE', *, *, #6465, .F. ) ;
#2948=CYLINDRICAL_SURFACE ( 'NONE', #15654, 5.000000000000000888 ) ;
#2949=VERTEX_POINT ( 'NONE', #2015 ) ;
#2958=CARTESIAN_POINT ( 'NONE',  ( 2.576507258269559397, -7.499999999999741540, -13.18245040793293121 ) ) ;
#2980=ORIENTED_EDGE ( 'NONE', *, *, #15931, .T. ) ;
#3013=DIRECTION ( 'NONE',  ( 6.938893903907227392E-16, 0.000000000000000000, 1.000000000000000000 ) ) ;
#3030=CARTESIAN_POINT ( 'NONE',  ( -6.538348415311014072, 7.499999999999999112, -16.99999999999999645 ) ) ;
#3050=CARTESIAN_POINT ( 'NONE',  ( 6.279379834064825694, -3.098285787162885718, -12.00000000061317884 ) ) ;
#3068=ORIENTED_EDGE ( 'NONE', *, *, #16880, .T. ) ;
#3073=CARTESIAN_POINT ( 'NONE',  ( -2.179449471770337432, -4.500000000000000000, 0.000000000000000000 ) ) ;
#3074=EDGE_LOOP ( 'NONE', ( #17384, #8165, #2527, #2937 ) ) ;
#3112=FACE_OUTER_BOUND ( 'NONE', #14632, .T. ) ;
#3130=CARTESIAN_POINT ( 'NONE',  ( -6.238556470687012911, 7.499999999999999112, -16.99999999974153297 ) ) ;
#3139=LINE ( 'NONE', #1928, #16071 ) ;
#3146=CARTESIAN_POINT ( 'NONE',  ( -20.00000000000000000, 2.499999999999998668, -12.00000000000000000 ) ) ;
#3147=CARTESIAN_POINT ( 'NONE',  ( 6.344274892086337658, -2.961199469785586125, -11.99999999981462295 ) ) ;
#3156=AXIS2_PLACEMENT_3D ( 'NONE', #11084, #16899, #5053 ) ;
#3185=VECTOR ( 'NONE', #6992, 1000.000000000000000 ) ;
#3194=ORIENTED_EDGE ( 'NONE', *, *, #744, .T. ) ;
#3197=CARTESIAN_POINT ( 'NONE',  ( -20.00000000000000000, -2.500000000000000444, -17.00000000000000000 ) ) ;
#3215=AXIS2_PLACEMENT_3D ( 'NONE', #3879, #828, #9981 ) ;
#3227=CARTESIAN_POINT ( 'NONE',  ( -3.381675179273344600, 7.499999999999998224, -16.15172605159659014 ) ) ;
#3240=EDGE_CURVE ( 'NONE', #5247, #15077, #10367, .T. ) ;
#3250=CARTESIAN_POINT ( 'NONE',  ( 2.166051897650331792, -7.500000000000000000, -13.14980647003173253 ) ) ;
#3254=CIRCLE ( 'NONE', #13946, 5.000000000000000000 ) ;
#3269=ORIENTED_EDGE ( 'NONE', *, *, #16857, .F. ) ;
#3293=VECTOR ( 'NONE', #11276, 1000.000000000000000 ) ;
#3316=ORIENTED_EDGE ( 'NONE', *, *, #10293, .F. ) ;
#3322=CARTESIAN_POINT ( 'NONE',  ( -20.00000000000000000, 2.499999999999998668, -17.00000000000000000 ) ) ;
#3330=CARTESIAN_POINT ( 'NONE',  ( 3.337222544067826480, 7.500000000000000000, -16.12749921823413146 ) ) ;
#3349=CARTESIAN_POINT ( 'NONE',  ( -1.329448181772147075, -7.499999999999999112, -13.08538760542149326 ) ) ;
#3369=ORIENTED_EDGE ( 'NONE', *, *, #14505, .F. ) ;
#3382=FILL_AREA_STYLE_COLOUR ( '', #12096 ) ;
#3383=DIRECTION ( 'NONE',  ( 0.8571673007021134438, 0.000000000000000000, 0.5150380749100522682 ) ) ;
#3390=FACE_OUTER_BOUND ( 'NONE', #12224, .T. ) ;
#3410=EDGE_CURVE ( 'NONE', #17372, #16531, #14936, .T. ) ;
#3413=DIRECTION ( 'NONE',  ( 0.000000000000000000, 0.000000000000000000, -1.000000000000000000 ) ) ;
#3429=CARTESIAN_POINT ( 'NONE',  ( -2.611994420159492680, 7.499999999999999112, -15.68429332095033146 ) ) ;
#3432=( NAMED_UNIT ( * ) SI_UNIT ( $, .STERADIAN. ) SOLID_ANGLE_UNIT ( ) );
#3447=CARTESIAN_POINT ( 'NONE',  ( -1.334466156054568975, -7.500000000000000888, -14.76217096505567383 ) ) ;
#3455=AXIS2_PLACEMENT_3D ( 'NONE', #876, #6894, #6994 ) ;
#3494=VERTEX_POINT ( 'NONE', #3984 ) ;
#3496=ORIENTED_EDGE ( 'NONE', *, *, #16309, .T. ) ;
#3501=CARTESIAN_POINT ( 'NONE',  ( 2.611515231136700699, -7.500000000000001776, -15.68397129924701439 ) ) ;
#3525=DIRECTION ( 'NONE',  ( -0.000000000000000000, 1.000000000000000000, -0.000000000000000000 ) ) ;
#3530=CARTESIAN_POINT ( 'NONE',  ( -6.021941181548490007, 3.575661417669479647, -12.00000000127642430 ) ) ;
#3545=CARTESIAN_POINT ( 'NONE',  ( 0.5390158121842351102, -6.982261029182121881, -11.99999999709518583 ) ) ;
#3569=VECTOR ( 'NONE', #7621, 1000.000000000000000 ) ;
#3615=DIRECTION ( 'NONE',  ( 0.000000000000000000, -0.000000000000000000, 1.000000000000000000 ) ) ;
#3625=CARTESIAN_POINT ( 'NONE',  ( -4.576598828870857005, 7.499999999999742428, -13.14213029402346500 ) ) ;
#3628=SURFACE_STYLE_FILL_AREA ( #16729 ) ;
#3639=CARTESIAN_POINT ( 'NONE',  ( -5.031681560115461416, -4.880796135282130521, -12.00000000472807926 ) ) ;
#3641=DIRECTION ( 'NONE',  ( 0.000000000000000000, -1.734723475976806848E-16, 1.000000000000000000 ) ) ;
#3679=DIRECTION ( 'NONE',  ( 1.000000000000000000, 0.000000000000000000, 0.000000000000000000 ) ) ;
#3687=CARTESIAN_POINT ( 'NONE',  ( -0.1112489676725734455, -7.500000000000002665, -14.17494330110305256 ) ) ;
#3706=VECTOR ( 'NONE', #14549, 1000.000000000000000 ) ;
#3715=CARTESIAN_POINT ( 'NONE',  ( 0.2633197948918147846, 7.499999999999999112, -14.20553286501796997 ) ) ;
#3729=CARTESIAN_POINT ( 'NONE',  ( 7.000000000000000000, 0.000000000000000000, 0.000000000000000000 ) ) ;
#3730=CARTESIAN_POINT ( 'NONE',  ( -0.6549932209174553766, -7.499999999999867661, -13.04593603512842037 ) ) ;
#3732=DIRECTION ( 'NONE',  ( -1.000000000000000000, 0.000000000000000000, 0.000000000000000000 ) ) ;
#3753=ORIENTED_EDGE ( 'NONE', *, *, #9599, .T. ) ;
#3760=CARTESIAN_POINT ( 'NONE',  ( -20.00000000000000000, -2.500000000000000444, -17.00000000000000000 ) ) ;
#3767=EDGE_CURVE ( 'NONE', #2949, #8066, #7293, .T. ) ;
#3778=CARTESIAN_POINT ( 'NONE',  ( 1.391363329066504617, -7.500000000000002665, -14.80343650618309503 ) ) ;
#3779=EDGE_CURVE ( 'NONE', #1187, #11848, #7386, .T. ) ;
#3806=CARTESIAN_POINT ( 'NONE',  ( -4.294575106066828241, 7.499999999999730882, -13.17881115347107901 ) ) ;
#3816=CARTESIAN_POINT ( 'NONE',  ( -20.00000000000000000, 2.499999999999998668, -22.00000000000000000 ) ) ;
#3831=VECTOR ( 'NONE', #2174, 1000.000000000000000 ) ;
#3838=ORIENTED_EDGE ( 'NONE', *, *, #17337, .T. ) ;
#3854=CIRCLE ( 'NONE', #6899, 5.000000000000000888 ) ;
#3860=DIRECTION ( 'NONE',  ( 0.000000000000000000, -0.000000000000000000, 1.000000000000000000 ) ) ;
#3879=CARTESIAN_POINT ( 'NONE',  ( 0.000000000000000000, -2.500000000000000444, -16.99999999999999645 ) ) ;
#3880=AXIS2_PLACEMENT_3D ( 'NONE', #1268, #18571, #5476 ) ;
#3903=CARTESIAN_POINT ( 'NONE',  ( 1.070106460717605401, 7.499999999999933387, -13.06798451319513532 ) ) ;
#3924=DIRECTION ( 'NONE',  ( 0.000000000000000000, 0.000000000000000000, -1.000000000000000000 ) ) ;
#3941=CARTESIAN_POINT ( 'NONE',  ( 6.538348415311010520, 2.499999999999998668, -12.00000000000000000 ) ) ;
#3946=DIRECTION ( 'NONE',  ( 1.000000000000000000, 0.000000000000000000, 0.000000000000000000 ) ) ;
#3965=DIRECTION ( 'NONE',  ( 0.000000000000000000, -0.000000000000000000, 1.000000000000000000 ) ) ;
#3984=CARTESIAN_POINT ( 'NONE',  ( 6.538348415311014072, -7.500000000000000888, -16.99999999999999645 ) ) ;
#3987=DIRECTION ( 'NONE',  ( -1.000000000000000000, 0.000000000000000000, 0.000000000000000000 ) ) ;
#3992=CARTESIAN_POINT ( 'NONE',  ( 5.029793280284322599, 7.499999999999999112, -16.81208494724229396 ) ) ;
#4007=CARTESIAN_POINT ( 'NONE',  ( -6.144877202871137811, -7.499999999999999112, -12.52666336607935094 ) ) ;
#4072=ORIENTED_EDGE ( 'NONE', *, *, #8028, .T. ) ;
#4081=FACE_OUTER_BOUND ( 'NONE', #8018, .T. ) ;
#4092=PLANE ( 'NONE',  #226 ) ;
#4097=EDGE_CURVE ( 'NONE', #16458, #13316, #16307, .T. ) ;
#4104=DIRECTION ( 'NONE',  ( -0.000000000000000000, 0.000000000000000000, -1.000000000000000000 ) ) ;
#4127=AXIS2_PLACEMENT_3D ( 'NONE', #5076, #12438, #10928 ) ;
#4153=EDGE_CURVE ( 'NONE', #18897, #5848, #15074, .T. ) ;
#4154=VERTEX_POINT ( 'NONE', #11946 ) ;
#4161=DIRECTION ( 'NONE',  ( 0.000000000000000000, -1.000000000000000000, -0.000000000000000000 ) ) ;
#4162=CYLINDRICAL_SURFACE ( 'NONE', #3215, 5.000000000000000888 ) ;
#4176=ORIENTED_EDGE ( 'NONE', *, *, #12342, .F. ) ;
#4188=CARTESIAN_POINT ( 'NONE',  ( 2.564349062531208645, 7.499999999999999112, -15.65236830614206909 ) ) ;
#4235=ADVANCED_FACE ( 'NONE', ( #9364 ), #11851, .T. ) ;
#4271=ORIENTED_EDGE ( 'NONE', *, *, #10896, .F. ) ;
#4278=CARTESIAN_POINT ( 'NONE',  ( 4.482738663876791207, 5.389345431477718940, -11.99999999527195627 ) ) ;
#4284=ADVANCED_FACE ( 'NONE', ( #483 ), #6310, .T. ) ;
#4314=CARTESIAN_POINT ( 'NONE',  ( -2.179449471770337432, -4.500000000000000000, -3.000000000000000000 ) ) ;
#4319=CARTESIAN_POINT ( 'NONE',  ( 1.876333640634852307, -7.500000000000000888, -15.16052078710814932 ) ) ;
#4332=ORIENTED_EDGE ( 'NONE', *, *, #3767, .T. ) ;
#4337=EDGE_CURVE ( 'NONE', #3494, #9678, #13853, .T. ) ;
#4364=CARTESIAN_POINT ( 'NONE',  ( 20.00000000000000000, 7.499999999999999112, -16.99999999999999645 ) ) ;
#4389=CYLINDRICAL_SURFACE ( 'NONE', #6098, 5.000000000000000888 ) ;
#4395=ORIENTED_EDGE ( 'NONE', *, *, #4153, .T. ) ;
#4405=CARTESIAN_POINT ( 'NONE',  ( 3.382406833283068348, -7.500000000000000888, -16.15212677409162012 ) ) ;
#4429=EDGE_LOOP ( 'NONE', ( #11404, #253, #4913, #370 ) ) ;
#4450=CARTESIAN_POINT ( 'NONE',  ( -20.00000000000000000, 0.000000000000000000, -22.00000000000000000 ) ) ;
#4463=LINE ( 'NONE', #4753, #12953 ) ;
#4496=CIRCLE ( 'NONE', #1123, 5.000000000000000888 ) ;
#4513=CARTESIAN_POINT ( 'NONE',  ( 6.439472576468413756, -7.500000000000131450, -12.20506288372488690 ) ) ;
#4551=CARTESIAN_POINT ( 'NONE',  ( 0.000000000000000000, 0.000000000000000000, -3.000000000000000000 ) ) ;
#4563=DIRECTION ( 'NONE',  ( 0.000000000000000000, 1.000000000000000000, 0.000000000000000000 ) ) ;
#4588=CARTESIAN_POINT ( 'NONE',  ( -2.863953186090931524, 7.500000000000000888, -15.84864299207352012 ) ) ;
#4605=CARTESIAN_POINT ( 'NONE',  ( 5.075684663107828065, -4.834325206103392780, -12.00000000445688464 ) ) ;
#4646=VECTOR ( 'NONE', #2672, 1000.000000000000000 ) ;
#4657=CARTESIAN_POINT ( 'NONE',  ( 20.00000000000000000, 2.499999999999998668, -17.00000000000000000 ) ) ;
#4698=AXIS2_PLACEMENT_3D ( 'NONE', #3197, #17551, #1499 ) ;
#4753=CARTESIAN_POINT ( 'NONE',  ( -25.00000000000000000, -7.500000000000000888, -16.99999999999999645 ) ) ;
#4766=VERTEX_POINT ( 'NONE', #7168 ) ;
#4798=CARTESIAN_POINT ( 'NONE',  ( -2.067729357296066883, -7.500000000000000888, -15.30380495029759480 ) ) ;
#4821=ORIENTED_EDGE ( 'NONE', *, *, #17337, .F. ) ;
#4877=DIRECTION ( 'NONE',  ( -0.000000000000000000, -0.000000000000000000, 1.000000000000000000 ) ) ;
#4880=CARTESIAN_POINT ( 'NONE',  ( -3.648056509801823388, 7.499999999999999112, -16.29094785500086573 ) ) ;
#4891=LINE ( 'NONE', #1829, #18513 ) ;
#4896=CARTESIAN_POINT ( 'NONE',  ( 0.4158217634471226276, -7.500000000000000888, -14.24727159067851368 ) ) ;
#4913=ORIENTED_EDGE ( 'NONE', *, *, #12538, .T. ) ;
#4918=EDGE_LOOP ( 'NONE', ( #4072, #4395, #2809 ) ) ;
#4919=CARTESIAN_POINT ( 'NONE',  ( -25.00000000000000000, 2.499999999999998668, -12.00000000000000000 ) ) ;
#4943=CARTESIAN_POINT ( 'NONE',  ( 5.051325721637065058, -7.500000000000001776, -16.81741242948696069 ) ) ;
#4953=ORIENTED_EDGE ( 'NONE', *, *, #14024, .T. ) ;
#4955=EDGE_LOOP ( 'NONE', ( #3194, #9210, #15704, #1357 ) ) ;
#4965=CARTESIAN_POINT ( 'NONE',  ( 0.2640320147533095074, 7.499999999999999112, -14.20017596028258744 ) ) ;
#4968=CARTESIAN_POINT ( 'NONE',  ( -0.3753471441346316051, 7.500000000000331291, -13.03644311608527850 ) ) ;
#4972=CARTESIAN_POINT ( 'NONE',  ( 2.179449471770337432, -4.500000000000000000, 0.000000000000000000 ) ) ;
#4978=ORIENTED_EDGE ( 'NONE', *, *, #11215, .F. ) ;
#4980=CARTESIAN_POINT ( 'NONE',  ( 1.149970134828444124, -6.907561563897677281, -11.99999999384792915 ) ) ;
#5005=AXIS2_PLACEMENT_3D ( 'NONE', #582, #289, #189 ) ;
#5027=CARTESIAN_POINT ( 'NONE',  ( 5.934112841479999290, -7.500000000000002665, -16.97589560338757408 ) ) ;
#5053=DIRECTION ( 'NONE',  ( -6.938893903907227392E-16, 0.000000000000000000, 1.000000000000000000 ) ) ;
#5055=CARTESIAN_POINT ( 'NONE',  ( 0.2197594725759999534, 7.500000000000027534, -13.03330426732994951 ) ) ;
#5070=CARTESIAN_POINT ( 'NONE',  ( -2.482385025457884087, -7.500000000000001776, -13.17615586950463857 ) ) ;
#5076=CARTESIAN_POINT ( 'NONE',  ( 20.00000000000000000, -2.500000000000000444, -17.00000000000000000 ) ) ;
#5123=EDGE_CURVE ( 'NONE', #15077, #5247, #8371, .T. ) ;
#5125=CARTESIAN_POINT ( 'NONE',  ( 1.876079424475004975, -7.500000000000001776, -15.16033210860608804 ) ) ;
#5128=DIRECTION ( 'NONE',  ( 0.000000000000000000, 0.000000000000000000, 1.000000000000000000 ) ) ;
#5139=ORIENTED_EDGE ( 'NONE', *, *, #14975, .T. ) ;
#5147=CARTESIAN_POINT ( 'NONE',  ( -6.154177238272306560, 7.499999999999997335, -12.51861270110133262 ) ) ;
#5151=CARTESIAN_POINT ( 'NONE',  ( 25.00000000000000000, -2.500000000000000444, -17.00000000000000000 ) ) ;
#5164=CARTESIAN_POINT ( 'NONE',  ( -0.4829358362134061333, -7.500000000000000888, -14.27056707468136665 ) ) ;
#5167=CYLINDRICAL_SURFACE ( 'NONE', #17229, 5.000000000000000888 ) ;
#5170=CARTESIAN_POINT ( 'NONE',  ( 6.538348415311010520, -2.500000000000000444, -12.00000000000000000 ) ) ;
#5191=CYLINDRICAL_SURFACE ( 'NONE', #6126, 7.000000000000000000 ) ;
#5216=CARTESIAN_POINT ( 'NONE',  ( -1.823557580623804908, -7.500000000000002665, -15.12114310604040845 ) ) ;
#5241=CARTESIAN_POINT ( 'NONE',  ( -1.213280723412490714, 7.499999999999931610, -13.07603167631473440 ) ) ;
#5246=CARTESIAN_POINT ( 'NONE',  ( 25.00000000000000000, -7.500000000000000888, -16.99999999999999645 ) ) ;
#5247=VERTEX_POINT ( 'NONE', #13782 ) ;
#5290=EDGE_CURVE ( 'NONE', #18780, #18879, #12118, .T. ) ;
#5294=LINE ( 'NONE', #2691, #15474 ) ;
#5303=CARTESIAN_POINT ( 'NONE',  ( 0.7623231285407791047, -7.500000000000001776, -14.39641017501655718 ) ) ;
#5309=AXIS2_PLACEMENT_3D ( 'NONE', #11179, #5599, #1027 ) ;
#5332=CARTESIAN_POINT ( 'NONE',  ( 6.499600586847153139, 2.601338725571119337, -12.00000000000000000 ) ) ;
#5339=AXIS2_PLACEMENT_3D ( 'NONE', #3760, #16584, #15418 ) ;
#5348=ORIENTED_EDGE ( 'NONE', *, *, #18195, .F. ) ;
#5349=DIRECTION ( 'NONE',  ( 0.000000000000000000, 0.000000000000000000, -1.000000000000000000 ) ) ;
#5350=CARTESIAN_POINT ( 'NONE',  ( -6.340401435272320363, -2.969608215370683979, -11.99999999980919618 ) ) ;
#5367=CARTESIAN_POINT ( 'NONE',  ( -6.538348415311010520, 2.499999999999998668, -12.00000000000000000 ) ) ;
#5401=DIRECTION ( 'NONE',  ( -1.000000000000000000, 0.000000000000000000, 0.000000000000000000 ) ) ;
#5419=EDGE_CURVE ( 'NONE', #5896, #1187, #3254, .T. ) ;
#5423=CARTESIAN_POINT ( 'NONE',  ( 4.153045036174358273, 5.656186534233338392, -12.00000000830655367 ) ) ;
#5426=CIRCLE ( 'NONE', #10306, 5.000000000000000888 ) ;
#5441=CARTESIAN_POINT ( 'NONE',  ( -6.259160902251362124, -7.500000000000261124, -12.42139992667873649 ) ) ;
#5453=DIRECTION ( 'NONE',  ( -1.000000000000000000, -0.000000000000000000, -0.000000000000000000 ) ) ;
#5476=DIRECTION ( 'NONE',  ( 0.000000000000000000, 0.000000000000000000, 1.000000000000000000 ) ) ;
#5503=DIRECTION ( 'NONE',  ( 0.000000000000000000, 0.000000000000000000, 1.000000000000000000 ) ) ;
#5507=CARTESIAN_POINT ( 'NONE',  ( 6.234321419756527760, 7.499999999999999112, -16.99999999998787104 ) ) ;
#5524=CARTESIAN_POINT ( 'NONE',  ( -6.273991221456290290, -3.109390318170350387, -12.00000000063440098 ) ) ;
#5549=DIRECTION ( 'NONE',  ( -0.000000000000000000, 0.000000000000000000, -1.000000000000000000 ) ) ;
#5557=CYLINDRICAL_SURFACE ( 'NONE', #3880, 5.000000000000000888 ) ;
#5561=ADVANCED_BREP_SHAPE_REPRESENTATION ( '', ( #10500, #2030 ), #9034 ) ;
#5563=EDGE_CURVE ( 'NONE', #12162, #8069, #3139, .T. ) ;
#5596=CARTESIAN_POINT ( 'NONE',  ( 5.045697689580606493, 7.500000000000000888, -13.04808138403512885 ) ) ;
#5598=LINE ( 'NONE', #11449, #9339 ) ;
#5599=DIRECTION ( 'NONE',  ( 0.000000000000000000, 0.000000000000000000, -1.000000000000000000 ) ) ;
#5617=EDGE_LOOP ( 'NONE', ( #18004, #16089 ) ) ;
#5691=CARTESIAN_POINT ( 'NONE',  ( 0.5544330523544508393, 7.499999999999999112, -14.29923508549706135 ) ) ;
#5701=VERTEX_POINT ( 'NONE', #3816 ) ;
#5752=EDGE_LOOP ( 'NONE', ( #10118, #4271, #15821 ) ) ;
#5760=ORIENTED_EDGE ( 'NONE', *, *, #12471, .T. ) ;
#5765=AXIS2_PLACEMENT_3D ( 'NONE', #11077, #3525, #15455 ) ;
#5768=LINE ( 'NONE', #8746, #11390 ) ;
#5803=ADVANCED_FACE ( 'NONE', ( #6977 ), #4092, .F. ) ;
#5818=VERTEX_POINT ( 'NONE', #15157 ) ;
#5830=CARTESIAN_POINT ( 'NONE',  ( 6.118503526523853431, -3.404981712889560974, -11.99999999938682294 ) ) ;
#5836=CARTESIAN_POINT ( 'NONE',  ( -2.500000000000000000, 3.061616997868383141E-16, -13.00000000000000533 ) ) ;
#5846=PLANE ( 'NONE',  #15780 ) ;
#5848=VERTEX_POINT ( 'NONE', #12005 ) ;
#5849=ORIENTED_EDGE ( 'NONE', *, *, #8215, .F. ) ;
#5852=DIRECTION ( 'NONE',  ( -1.000000000000000000, 0.000000000000000000, 0.000000000000000000 ) ) ;
#5883=ADVANCED_FACE ( 'NONE', ( #3390 ), #6078, .F. ) ;
#5896=VERTEX_POINT ( 'NONE', #15430 ) ;
#5908=DIRECTION ( 'NONE',  ( 1.000000000000000000, 0.000000000000000000, -0.000000000000000000 ) ) ;
#5909=ADVANCED_FACE ( 'NONE', ( #724, #11137 ), #12468, .F. ) ;
#5946=ORIENTED_EDGE ( 'NONE', *, *, #13616, .T. ) ;
#5951=VECTOR ( 'NONE', #7364, 1000.000000000000000 ) ;
#6004=ADVANCED_FACE ( 'NONE', ( #11051 ), #12287, .T. ) ;
#6005=AXIS2_PLACEMENT_3D ( 'NONE', #12810, #5453, #7185 ) ;
#6027=VECTOR ( 'NONE', #7888, 1000.000000000000000 ) ;
#6041=CARTESIAN_POINT ( 'NONE',  ( 5.872941918983158871, -7.500000000000001776, -12.71526091932864766 ) ) ;
#6075=CARTESIAN_POINT ( 'NONE',  ( 25.00000000000000000, -2.500000000000000444, -16.99999999999999645 ) ) ;
#6078=CYLINDRICAL_SURFACE ( 'NONE', #13346, 2.500000000000000000 ) ;
#6093=ADVANCED_FACE ( 'NONE', ( #9864 ), #5846, .T. ) ;
#6098=AXIS2_PLACEMENT_3D ( 'NONE', #10220, #9079, #7369 ) ;
#6126=AXIS2_PLACEMENT_3D ( 'NONE', #16672, #2232, #3946 ) ;
#6137=CARTESIAN_POINT ( 'NONE',  ( 3.329573251200529160, -7.500000000000264677, -13.21489263293670469 ) ) ;
#6194=ORIENTED_EDGE ( 'NONE', *, *, #12538, .F. ) ;
#6228=CARTESIAN_POINT ( 'NONE',  ( -1.517261107235201356, -6.836011689345085962, -11.99999999467221912 ) ) ;
#6245=EDGE_LOOP ( 'NONE', ( #12307, #15035 ) ) ;
#6255=EDGE_LOOP ( 'NONE', ( #2692, #11300 ) ) ;
#6264=( LENGTH_UNIT ( ) NAMED_UNIT ( * ) SI_UNIT ( .MILLI., .METRE. ) );
#6266=DIRECTION ( 'NONE',  ( 2.081668171172168119E-15, 0.000000000000000000, 1.000000000000000000 ) ) ;
#6298=AXIS2_PLACEMENT_3D ( 'NONE', #16894, #9722, #9629 ) ;
#6309=CARTESIAN_POINT ( 'NONE',  ( -5.051325721637062394, 7.500000000000000000, -16.81741242948696069 ) ) ;
#6310=CYLINDRICAL_SURFACE ( 'NONE', #10182, 7.000000000000000000 ) ;
#6311=CARTESIAN_POINT ( 'NONE',  ( -6.118503526524619041, 3.404981712888209611, -11.99999999938683892 ) ) ;
#6332=CARTESIAN_POINT ( 'NONE',  ( 0.2286586286997084050, -7.499999999999928946, -13.03338879287354679 ) ) ;
#6336=AXIS2_PLACEMENT_3D ( 'NONE', #11237, #12649, #8000 ) ;
#6368=SURFACE_SIDE_STYLE ('',( #15241 ) ) ;
#6378=VERTEX_POINT ( 'NONE', #5367 ) ;
#6383=FACE_OUTER_BOUND ( 'NONE', #12085, .T. ) ;
#6388=LINE ( 'NONE', #14010, #3831 ) ;
#6408=CARTESIAN_POINT ( 'NONE',  ( -5.704021078596165140, 7.500000000000000000, -12.80826310103332943 ) ) ;
#6412=DIRECTION ( 'NONE',  ( 0.000000000000000000, -1.000000000000000000, 0.000000000000000000 ) ) ;
#6425=CARTESIAN_POINT ( 'NONE',  ( 0.3753471441347580040, -7.499999999999771738, -13.03644311608535133 ) ) ;
#6463=B_SPLINE_CURVE_WITH_KNOTS ( 'NONE', 3,
 ( #9606, #12477, #5027, #13909, #4943, #18126, #823, #10968, #6664, #10774, #3501, #15342, #5125, #3778, #13733, #5303, #16788, #15258, #16875, #3687, #10878, #9518, #12566, #2253, #18309, #5216, #11057, #2431, #15437, #8190, #14007, #915, #9341, #6755, #18219, #9703, #16696, #2086 ),
 .UNSPECIFIED., .F., .F.,
 ( 4, 2, 2, 2, 2, 2, 2, 2, 2, 2, 2, 2, 2, 2, 2, 2, 2, 2, 4 ),
 ( 0.000000000000000000, 0.0009058109605214382685, 0.001811621921042876537, 0.002717432881564314697, 0.003623243842085754375, 0.004529054802607194487, 0.005434865763128634598, 0.006340676723650073843, 0.006793582203910795633, 0.007246487684171517424, 0.007699393164432237480, 0.008152298644692957535, 0.009058109605214399382, 0.009963920565735841228, 0.01086973152625728307, 0.01177554248677872319, 0.01268135344730016677, 0.01358716440782160688, 0.01449297536834305046 ),
 .UNSPECIFIED. ) ;
#6465=EDGE_CURVE ( 'NONE', #5896, #7194, #15585, .T. ) ;
#6500=CARTESIAN_POINT ( 'NONE',  ( 0.06860918897775840353, 7.499999999999997335, -13.03178490627139219 ) ) ;
#6513=AXIS2_PLACEMENT_3D ( 'NONE', #1773, #1669, #15910 ) ;
#6517=CARTESIAN_POINT ( 'NONE',  ( -0.5119965487699434936, -7.500000000000230926, -13.04039602617929638 ) ) ;
#6550=SHAPE_REPRESENTATION_RELATIONSHIP ( 'NONE' , 'NONE' ,  #11674, #5561 ) ;
#6581=EDGE_LOOP ( 'NONE', ( #158, #3068, #15724, #16261 ) ) ;
#6592=CARTESIAN_POINT ( 'NONE',  ( 0.1127451301831694647, 7.499999999999999112, -14.18240585847532742 ) ) ;
#6606=ORIENTED_EDGE ( 'NONE', *, *, #3410, .F. ) ;
#6610=CARTESIAN_POINT ( 'NONE',  ( -5.045697689581268186, -7.500000000000132339, -13.04808138403488549 ) ) ;
#6612=CARTESIAN_POINT ( 'NONE',  ( 25.00000000000000000, -2.500000000000000444, -12.00000000000000000 ) ) ;
#6628=AXIS2_PLACEMENT_3D ( 'NONE', #14467, #5401, #1379 ) ;
#6664=CARTESIAN_POINT ( 'NONE',  ( 3.381675179273347265, -7.500000000000001776, -16.15172605159659369 ) ) ;
#6675=ORIENTED_EDGE ( 'NONE', *, *, #15896, .F. ) ;
#6688=CARTESIAN_POINT ( 'NONE',  ( -3.382406833283016390, 7.499999999999999112, -16.15212677409211040 ) ) ;
#6699=CIRCLE ( 'NONE', #12483, 2.500000000000000000 ) ;
#6731=EDGE_CURVE ( 'NONE', #8559, #12766, #8304, .T. ) ;
#6755=CARTESIAN_POINT ( 'NONE',  ( -5.027901255400313296, -7.500000000000000888, -16.81159201184369323 ) ) ;
#6768=ORIENTED_EDGE ( 'NONE', *, *, #12471, .F. ) ;
#6775=CYLINDRICAL_SURFACE ( 'NONE', #13951, 5.000000000000000000 ) ;
#6779=CARTESIAN_POINT ( 'NONE',  ( 3.601232060344256247, 7.499999999999740652, -13.21583132166216679 ) ) ;
#6851=ADVANCED_FACE ( 'NONE', ( #11934 ), #9357, .T. ) ;
#6852=EDGE_LOOP ( 'NONE', ( #8991, #17405, #1392, #3496 ) ) ;
#6865=CARTESIAN_POINT ( 'NONE',  ( 6.108979705494776979, 3.422227477007715013, -11.99999999936562567 ) ) ;
#6879=DIRECTION ( 'NONE',  ( -1.000000000000000000, 0.000000000000000000, 0.000000000000000000 ) ) ;
#6884=CARTESIAN_POINT ( 'NONE',  ( 20.00000000000000000, 2.499999999999997780, -16.99999999999999645 ) ) ;
#6890=CYLINDRICAL_SURFACE ( 'NONE', #2873, 5.000000000000000888 ) ;
#6894=DIRECTION ( 'NONE',  ( -1.000000000000000000, -0.000000000000000000, -0.000000000000000000 ) ) ;
#6899=AXIS2_PLACEMENT_3D ( 'NONE', #8366, #13036, #11608 ) ;
#6963=CARTESIAN_POINT ( 'NONE',  ( 0.000000000000000000, 0.000000000000000000, 0.000000000000000000 ) ) ;
#6967=CARTESIAN_POINT ( 'NONE',  ( 1.329448181772381776, 7.500000000000063949, -13.08538760542143464 ) ) ;
#6974=DIRECTION ( 'NONE',  ( 0.000000000000000000, 0.000000000000000000, -1.000000000000000000 ) ) ;
#6977=FACE_OUTER_BOUND ( 'NONE', #9251, .T. ) ;
#6984=CARTESIAN_POINT ( 'NONE',  ( -6.538348415310987427, -2.500000000000060396, -12.00000000000000000 ) ) ;
#6988=FACE_OUTER_BOUND ( 'NONE', #13385, .T. ) ;
#6992=DIRECTION ( 'NONE',  ( -0.000000000000000000, -0.000000000000000000, 1.000000000000000000 ) ) ;
#6994=DIRECTION ( 'NONE',  ( 0.000000000000000000, 8.673617379884033500E-16, -1.000000000000000000 ) ) ;
#7017=DIRECTION ( 'NONE',  ( -0.000000000000000000, -1.000000000000000000, -0.000000000000000000 ) ) ;
#7042=ORIENTED_EDGE ( 'NONE', *, *, #18832, .T. ) ;
#7056=CARTESIAN_POINT ( 'NONE',  ( 1.334466156054132657, 7.499999999999999112, -14.76217096505626181 ) ) ;
#7071=DIRECTION ( 'NONE',  ( 1.000000000000000000, 0.000000000000000000, 0.000000000000000000 ) ) ;
#7077=CARTESIAN_POINT ( 'NONE',  ( 0.000000000000000000, 0.000000000000000000, -12.00000000000000000 ) ) ;
#7081=DIRECTION ( 'NONE',  ( 1.000000000000000000, 0.000000000000000000, 0.000000000000000000 ) ) ;
#7114=ORIENTED_EDGE ( 'NONE', *, *, #2377, .T. ) ;
#7131=CIRCLE ( 'NONE', #12602, 5.000000000000000888 ) ;
#7149=CARTESIAN_POINT ( 'NONE',  ( 0.7597029211760544243, 7.499999999999999112, -14.39758526244293790 ) ) ;
#7168=CARTESIAN_POINT ( 'NONE',  ( 20.00000000000000000, 2.499999999999998668, -12.00000000000000000 ) ) ;
#7170=ORIENTED_EDGE ( 'NONE', *, *, #13616, .F. ) ;
#7185=DIRECTION ( 'NONE',  ( 0.000000000000000000, 0.000000000000000000, -1.000000000000000000 ) ) ;
#7194=VERTEX_POINT ( 'NONE', #3073 ) ;
#7195=DIRECTION ( 'NONE',  ( -0.000000000000000000, -0.000000000000000000, 1.000000000000000000 ) ) ;
#7230=EDGE_CURVE ( 'NONE', #13316, #7194, #2883, .T. ) ;
#7264=ORIENTED_EDGE ( 'NONE', *, *, #9862, .T. ) ;
#7271=AXIS2_PLACEMENT_3D ( 'NONE', #10569, #437, #6266 ) ;
#7293=LINE ( 'NONE', #5836, #14620 ) ;
#7364=DIRECTION ( 'NONE',  ( -0.000000000000000000, -0.000000000000000000, 1.000000000000000000 ) ) ;
#7366=FACE_BOUND ( 'NONE', #6245, .T. ) ;
#7369=DIRECTION ( 'NONE',  ( 0.000000000000000000, 0.000000000000000000, -1.000000000000000000 ) ) ;
#7383=CARTESIAN_POINT ( 'NONE',  ( 1.715145640900883395, -6.797472175340068645, -12.00000001230414348 ) ) ;
#7386=LINE ( 'NONE', #13200, #16157 ) ;
#7403=ORIENTED_EDGE ( 'NONE', *, *, #16309, .F. ) ;
#7429=ORIENTED_EDGE ( 'NONE', *, *, #17630, .T. ) ;
#7460=CARTESIAN_POINT ( 'NONE',  ( 0.000000000000000000, 0.000000000000000000, -12.00000000000000000 ) ) ;
#7462=CARTESIAN_POINT ( 'NONE',  ( -0.6293707761309729198, 7.500000000000000000, -14.32724244806440161 ) ) ;
#7479=CARTESIAN_POINT ( 'NONE',  ( 4.196046169205040144, -7.500000000000000888, -16.53685941778015689 ) ) ;
#7485=DIRECTION ( 'NONE',  ( 1.000000000000000000, 0.000000000000000000, 0.000000000000000000 ) ) ;
#7499=ADVANCED_FACE ( 'NONE', ( #17502 ), #23, .T. ) ;
#7506=VERTEX_POINT ( 'NONE', #14052 ) ;
#7516=EDGE_CURVE ( 'NONE', #9395, #18705, #7796, .T. ) ;
#7531=DIRECTION ( 'NONE',  ( 0.000000000000000000, 0.000000000000000000, -1.000000000000000000 ) ) ;
#7545=DIRECTION ( 'NONE',  ( 0.000000000000000000, 0.000000000000000000, -1.000000000000000000 ) ) ;
#7562=CARTESIAN_POINT ( 'NONE',  ( -1.876079424475003199, 7.500000000000000000, -15.16033210860608804 ) ) ;
#7566=CARTESIAN_POINT ( 'NONE',  ( -6.439472576468937781, 7.500000000000000000, -12.20506288372541093 ) ) ;
#7582=VECTOR ( 'NONE', #465, 1000.000000000000000 ) ;
#7585=CARTESIAN_POINT ( 'NONE',  ( 5.704021078595903127, -7.499999999999735323, -12.80826310103411991 ) ) ;
#7603=ORIENTED_EDGE ( 'NONE', *, *, #3410, .T. ) ;
#7618=ADVANCED_FACE ( 'NONE', ( #16241 ), #10506, .F. ) ;
#7621=DIRECTION ( 'NONE',  ( 0.000000000000000000, 1.000000000000000000, 0.000000000000000000 ) ) ;
#7658=CARTESIAN_POINT ( 'NONE',  ( 0.5553368343811782015, 7.500000000000000000, -14.29382045140261503 ) ) ;
#7659=DIRECTION ( 'NONE',  ( 0.000000000000000000, 0.000000000000000000, -1.000000000000000000 ) ) ;
#7660=CARTESIAN_POINT ( 'NONE',  ( -20.00000000000000000, -2.500000000000000444, -16.99999999999999645 ) ) ;
#7664=AXIS2_PLACEMENT_3D ( 'NONE', #12821, #5549, #11399 ) ;
#7675=CARTESIAN_POINT ( 'NONE',  ( 1.149093537842186707, -7.500000000000000888, -14.62468756229394629 ) ) ;
#7693=ORIENTED_EDGE ( 'NONE', *, *, #7516, .F. ) ;
#7696=ORIENTED_EDGE ( 'NONE', *, *, #5290, .F. ) ;
#7702=ORIENTED_EDGE ( 'NONE', *, *, #17661, .T. ) ;
#7726=SPHERICAL_SURFACE ( 'NONE', #10204, 5.000000000000000000 ) ;
#7728=PRODUCT_DEFINITION_CONTEXT ( 'detailed design', #17804, 'design' ) ;
#7729=CARTESIAN_POINT ( 'NONE',  ( 0.000000000000000000, 0.000000000000000000, 0.000000000000000000 ) ) ;
#7751=CARTESIAN_POINT ( 'NONE',  ( 2.066926351139553475, 7.499999999999999112, -15.30321684074790056 ) ) ;
#7768=CARTESIAN_POINT ( 'NONE',  ( -0.2197594725757872069, -7.499999999999768185, -13.03330426733007386 ) ) ;
#7795=ORIENTED_EDGE ( 'NONE', *, *, #17118, .F. ) ;
#7796=CIRCLE ( 'NONE', #9597, 5.000000000000000000 ) ;
#7808=VECTOR ( 'NONE', #1939, 1000.000000000000000 ) ;
#7827=DIRECTION ( 'NONE',  ( -1.000000000000000000, 0.000000000000000000, 0.000000000000000000 ) ) ;
#7847=CARTESIAN_POINT ( 'NONE',  ( -4.195027931520234787, 7.500000000000000000, -16.53644619669688254 ) ) ;
#7850=CARTESIAN_POINT ( 'NONE',  ( -1.876333640634785693, 7.499999999999999112, -15.16052078710835715 ) ) ;
#7870=CARTESIAN_POINT ( 'NONE',  ( -0.06860918897761346391, -7.500000000000061284, -13.03178490627152186 ) ) ;
#7888=DIRECTION ( 'NONE',  ( -0.000000000000000000, -0.000000000000000000, 1.000000000000000000 ) ) ;
#7892=DIRECTION ( 'NONE',  ( -1.000000000000000000, 0.000000000000000000, 0.000000000000000000 ) ) ;
#7932=ORIENTED_EDGE ( 'NONE', *, *, #2463, .T. ) ;
#7950=CARTESIAN_POINT ( 'NONE',  ( -5.288115175735990547, 4.595214139557860733, -11.99999999743909740 ) ) ;
#7963=CARTESIAN_POINT ( 'NONE',  ( -3.324307330593659238, -6.179741886604213974, -11.99999999169353160 ) ) ;
#7999=VECTOR ( 'NONE', #2038, 1000.000000000000000 ) ;
#8000=DIRECTION ( 'NONE',  ( -1.000000000000000000, 0.000000000000000000, -0.000000000000000000 ) ) ;
#8018=EDGE_LOOP ( 'NONE', ( #10777, #14650, #16824, #16092 ) ) ;
#8028=EDGE_CURVE ( 'NONE', #622, #18897, #14194, .T. ) ;
#8035=CARTESIAN_POINT ( 'NONE',  ( -4.227723179941619058, 5.599337756632279728, -12.00000000790602428 ) ) ;
#8046=EDGE_CURVE ( 'NONE', #18780, #13920, #10862, .T. ) ;
#8051=CARTESIAN_POINT ( 'NONE',  ( -0.6925461861254285090, -7.500000000000000888, -14.36265820198516074 ) ) ;
#8066=VERTEX_POINT ( 'NONE', #8657 ) ;
#8069=VERTEX_POINT ( 'NONE', #4364 ) ;
#8077=PRODUCT_DEFINITION_FORMATION_WITH_SPECIFIED_SOURCE ( 'ANY', '', #684, .NOT_KNOWN. ) ;
#8106=FACE_OUTER_BOUND ( 'NONE', #13413, .T. ) ;
#8115=AXIS2_PLACEMENT_3D ( 'NONE', #16373, #16469, #7485 ) ;
#8126=CARTESIAN_POINT ( 'NONE',  ( -5.872941918984155407, 7.499999999999997335, -12.71526091932764224 ) ) ;
#8141=CARTESIAN_POINT ( 'NONE',  ( -3.606670283718027559, -7.500000000000000888, -16.27044756620548327 ) ) ;
#8165=ORIENTED_EDGE ( 'NONE', *, *, #3779, .T. ) ;
#8171=CLOSED_SHELL ( 'NONE', ( #13610, #1637, #16651, #2441, #4284, #6093, #16758, #5909, #17703, #5803, #14103, #8784, #15299, #4235, #18490, #2246, #14625, #14623, #1229, #1844, #7499, #10017, #11875, #17409, #13290, #6004, #2392, #2154, #9963, #9740, #1026, #17408, #7618, #6851, #1955, #5883, #9438 ) ) ;
#8176=EDGE_CURVE ( 'NONE', #9741, #748, #11469, .T. ) ;
#8188=DIRECTION ( 'NONE',  ( 1.000000000000000000, 0.000000000000000000, -0.000000000000000000 ) ) ;
#8190=CARTESIAN_POINT ( 'NONE',  ( -3.337222544067827368, -7.500000000000000888, -16.12749921823413146 ) ) ;
#8200=ORIENTED_EDGE ( 'NONE', *, *, #10608, .F. ) ;
#8215=EDGE_CURVE ( 'NONE', #1807, #6378, #1065, .T. ) ;
#8216=CARTESIAN_POINT ( 'NONE',  ( -6.279379834064045873, 3.098285787164263283, -12.00000000061316108 ) ) ;
#8221=CYLINDRICAL_SURFACE ( 'NONE', #14076, 5.000000000000000888 ) ;
#8279=SPHERICAL_SURFACE ( 'NONE', #15407, 5.000000000000000000 ) ;
#8292=ORIENTED_EDGE ( 'NONE', *, *, #14437, .F. ) ;
#8302=CARTESIAN_POINT ( 'NONE',  ( 4.449459268825830982, 7.499999999999999112, -16.63368482084348798 ) ) ;
#8304=CIRCLE ( 'NONE', #981, 5.000000000000000888 ) ;
#8323=DIRECTION ( 'NONE',  ( -1.000000000000000000, -0.000000000000000000, 0.000000000000000000 ) ) ;
#8366=CARTESIAN_POINT ( 'NONE',  ( -6.538348415311006967, 2.499999999999998668, -17.00000000000000000 ) ) ;
#8371=CIRCLE ( 'NONE', #13865, 2.500000000000000000 ) ;
#8379=CIRCLE ( 'NONE', #11213, 7.000000000000000000 ) ;
#8389=CARTESIAN_POINT ( 'NONE',  ( 0.6549932209177148357, 7.499999999999867661, -13.04593603512842570 ) ) ;
#8394=CARTESIAN_POINT ( 'NONE',  ( -6.538348415311014072, -7.500000000000000888, -16.99999999999999645 ) ) ;
#8397=CONICAL_SURFACE ( 'NONE', #8115, 2.500000000000000000, 1.029744258676656754 ) ;
#8404=ORIENTED_EDGE ( 'NONE', *, *, #4097, .F. ) ;
#8406=CARTESIAN_POINT ( 'NONE',  ( -6.234321419756340354, -7.500000000000000888, -16.99999999998787104 ) ) ;
#8415=LINE ( 'NONE', #14247, #3185 ) ;
#8434=UNCERTAINTY_MEASURE_WITH_UNIT (LENGTH_MEASURE( 1.000000000000000082E-05 ), #2113, 'distance_accuracy_value', 'NONE');
#8441=LINE ( 'NONE', #1179, #1959 ) ;
#8460=CARTESIAN_POINT ( 'NONE',  ( 0.000000000000000000, 0.000000000000000000, 0.000000000000000000 ) ) ;
#8464=CARTESIAN_POINT ( 'NONE',  ( -19.99999999999999645, 7.499999999999999112, -17.00000000000000000 ) ) ;
#8483=CARTESIAN_POINT ( 'NONE',  ( 2.817269318715503790, 7.499999999999999112, -15.81922481682711634 ) ) ;
#8485=EDGE_CURVE ( 'NONE', #8069, #12401, #1716, .T. ) ;
#8528=CIRCLE ( 'NONE', #2713, 5.000000000000000888 ) ;
#8559=VERTEX_POINT ( 'NONE', #9997 ) ;
#8573=CARTESIAN_POINT ( 'NONE',  ( 2.037104019874286465, 6.699095661347369557, -11.99999999578282406 ) ) ;
#8574=CARTESIAN_POINT ( 'NONE',  ( 0.000000000000000000, 0.000000000000000000, -3.000000000000000000 ) ) ;
#8591=DIRECTION ( 'NONE',  ( 0.000000000000000000, 0.000000000000000000, 1.000000000000000000 ) ) ;
#8598=FACE_OUTER_BOUND ( 'NONE', #105, .T. ) ;
#8609=ORIENTED_EDGE ( 'NONE', *, *, #14362, .T. ) ;
#8657=CARTESIAN_POINT ( 'NONE',  ( -2.500000000000000000, 3.061616997868383141E-16, -13.00000000000000533 ) ) ;
#8662=CARTESIAN_POINT ( 'NONE',  ( 6.340401435272480235, 2.969608215370613813, -11.99999999980921572 ) ) ;
#8664=DIRECTION ( 'NONE',  ( 1.000000000000000000, 0.000000000000000000, 0.000000000000000000 ) ) ;
#8684=CARTESIAN_POINT ( 'NONE',  ( 0.000000000000000000, 0.000000000000000000, 0.000000000000000000 ) ) ;
#8709=CARTESIAN_POINT ( 'NONE',  ( 5.783659440659287831, -3.949482697158031463, -11.99999999872349576 ) ) ;
#8746=CARTESIAN_POINT ( 'NONE',  ( 5.000000000000000000, 0.000000000000000000, 0.000000000000000000 ) ) ;
#8754=ORIENTED_EDGE ( 'NONE', *, *, #3240, .T. ) ;
#8784=ADVANCED_FACE ( 'NONE', ( #12658 ), #15341, .T. ) ;
#8789=EDGE_LOOP ( 'NONE', ( #3369, #232, #8200, #13923, #11668, #2123 ) ) ;
#8793=DIRECTION ( 'NONE',  ( 0.000000000000000000, 0.000000000000000000, -1.000000000000000000 ) ) ;
#8796=CARTESIAN_POINT ( 'NONE',  ( 0.000000000000000000, 2.499999999999998668, -16.99999999999999645 ) ) ;
#8805=CARTESIAN_POINT ( 'NONE',  ( 1.461502493107205369, -7.499999999999999112, -13.09494173305809817 ) ) ;
#8878=CARTESIAN_POINT ( 'NONE',  ( -2.117556820461446332, 7.500000000000000000, -15.34001259936770545 ) ) ;
#8883=DIRECTION ( 'NONE',  ( -1.000000000000000000, 0.000000000000000000, -1.335737076501871514E-14 ) ) ;
#8900=LINE ( 'NONE', #16172, #7808 ) ;
#8911=ORIENTED_EDGE ( 'NONE', *, *, #2465, .F. ) ;
#8917=EDGE_LOOP ( 'NONE', ( #128, #9718, #11986 ) ) ;
#8942=EDGE_CURVE ( 'NONE', #6378, #17649, #3854, .T. ) ;
#8954=CIRCLE ( 'NONE', #3455, 5.000000000000000888 ) ;
#8955=CIRCLE ( 'NONE', #4698, 5.000000000000000888 ) ;
#8968=AXIS2_PLACEMENT_3D ( 'NONE', #8976, #16348, #7659 ) ;
#8974=CARTESIAN_POINT ( 'NONE',  ( 0.6933513387705728670, 7.500000000000000888, -14.36029122898768939 ) ) ;
#8976=CARTESIAN_POINT ( 'NONE',  ( 20.00000000000000000, -2.500000000000000444, -17.00000000000000000 ) ) ;
#8991=ORIENTED_EDGE ( 'NONE', *, *, #2465, .T. ) ;
#9016=DIRECTION ( 'NONE',  ( 0.000000000000000000, 0.000000000000000000, -1.000000000000000000 ) ) ;
#9034=( GEOMETRIC_REPRESENTATION_CONTEXT ( 3 ) GLOBAL_UNCERTAINTY_ASSIGNED_CONTEXT ( ( #1736 ) ) GLOBAL_UNIT_ASSIGNED_CONTEXT ( ( #1576, #1772, #11999 ) ) REPRESENTATION_CONTEXT ( 'NONE', 'WORKASPACE' ) );
#9039=DIRECTION ( 'NONE',  ( 0.000000000000000000, 1.000000000000000000, 0.000000000000000000 ) ) ;
#9076=CARTESIAN_POINT ( 'NONE',  ( 2.816212223827430083, 7.499999999999999112, -15.81854889450411861 ) ) ;
#9079=DIRECTION ( 'NONE',  ( 0.000000000000000000, -1.000000000000000000, 0.000000000000000000 ) ) ;
#9096=CARTESIAN_POINT ( 'NONE',  ( 6.538348415311011408, -2.499999999999998668, -12.00000000000000000 ) ) ;
#9104=VECTOR ( 'NONE', #412, 1000.000000000000000 ) ;
#9169=CARTESIAN_POINT ( 'NONE',  ( 4.160991745704745171, 7.500000000000000888, -16.52287405655582475 ) ) ;
#9172=FACE_OUTER_BOUND ( 'NONE', #230, .T. ) ;
#9182=EDGE_CURVE ( 'NONE', #17372, #12766, #16980, .T. ) ;
#9186=CARTESIAN_POINT ( 'NONE',  ( -0.9342146476564506807, -7.500000000000132339, -13.05973490260134362 ) ) ;
#9210=ORIENTED_EDGE ( 'NONE', *, *, #11124, .T. ) ;
#9249=CIRCLE ( 'NONE', #6513, 5.000000000000000000 ) ;
#9251=EDGE_LOOP ( 'NONE', ( #8609, #7114 ) ) ;
#9266=CARTESIAN_POINT ( 'NONE',  ( -2.117882332753601826, 7.499999999999999112, -15.34025089741873238 ) ) ;
#9281=CARTESIAN_POINT ( 'NONE',  ( -2.817269318714846094, -7.500000000000000888, -15.81922481682703996 ) ) ;
#9339=VECTOR ( 'NONE', #17267, 1000.000000000000000 ) ;
#9341=CARTESIAN_POINT ( 'NONE',  ( -4.447775431366607357, -7.500000000000001776, -16.63307795419225954 ) ) ;
#9347=DIRECTION ( 'NONE',  ( -0.000000000000000000, -0.000000000000000000, 1.000000000000000000 ) ) ;
#9357=PLANE ( 'NONE',  #13796 ) ;
#9364=FACE_OUTER_BOUND ( 'NONE', #10658, .T. ) ;
#9365=CARTESIAN_POINT ( 'NONE',  ( -0.2286586286994273798, 7.499999999999998224, -13.03338879287367824 ) ) ;
#9385=CARTESIAN_POINT ( 'NONE',  ( -0.3372494957989286557, -7.500000000000000888, -14.22369192593361831 ) ) ;
#9390=LINE ( 'NONE', #11106, #1366 ) ;
#9395=VERTEX_POINT ( 'NONE', #2589 ) ;
#9418=ORIENTED_EDGE ( 'NONE', *, *, #11755, .F. ) ;
#9424=EDGE_CURVE ( 'NONE', #5701, #12401, #8900, .T. ) ;
#9438=ADVANCED_FACE ( 'NONE', ( #11679 ), #8397, .F. ) ;
#9461=CARTESIAN_POINT ( 'NONE',  ( -5.075684663107223216, 4.834325206103791572, -12.00000000445675319 ) ) ;
#9474=CARTESIAN_POINT ( 'NONE',  ( -5.250594443111816112, -4.638468187398823162, -11.99999999738842682 ) ) ;
#9487=LINE ( 'NONE', #2220, #6027 ) ;
#9512=EDGE_CURVE ( 'NONE', #12401, #18780, #9390, .T. ) ;
#9518=CARTESIAN_POINT ( 'NONE',  ( -0.5553368343811752039, -7.500000000000002665, -14.29382045140262036 ) ) ;
#9542=CARTESIAN_POINT ( 'NONE',  ( 0.9371186270715102795, 6.939831204821730104, -11.99999999628260561 ) ) ;
#9547=DIRECTION ( 'NONE',  ( 0.000000000000000000, 0.000000000000000000, -1.000000000000000000 ) ) ;
#9557=CARTESIAN_POINT ( 'NONE',  ( 0.000000000000000000, 0.000000000000000000, 0.000000000000000000 ) ) ;
#9558=CARTESIAN_POINT ( 'NONE',  ( -3.253466017772906227, -7.500000000000001776, -13.21345932477064444 ) ) ;
#9583=MECHANICAL_DESIGN_GEOMETRIC_PRESENTATION_REPRESENTATION('',(#17798),#15669);
#9597=AXIS2_PLACEMENT_3D ( 'NONE', #17102, #4104, #7071 ) ;
#9599=EDGE_CURVE ( 'NONE', #13920, #18879, #15423, .T. ) ;
#9603=ORIENTED_EDGE ( 'NONE', *, *, #5563, .T. ) ;
#9606=CARTESIAN_POINT ( 'NONE',  ( 6.538348415311014072, -7.500000000000000888, -16.99999999999999645 ) ) ;
#9619=EDGE_LOOP ( 'NONE', ( #183, #12396, #16288, #8911 ) ) ;
#9629=DIRECTION ( 'NONE',  ( 0.000000000000000000, 0.000000000000000000, -1.000000000000000000 ) ) ;
#9634=CARTESIAN_POINT ( 'NONE',  ( -0.3417098569969649335, 7.499999999999999112, -14.22469181348822431 ) ) ;
#9670=CIRCLE ( 'NONE', #6628, 5.000000000000000888 ) ;
#9678=VERTEX_POINT ( 'NONE', #5170 ) ;
#9701=CIRCLE ( 'NONE', #7271, 5.000000000000000888 ) ;
#9703=CARTESIAN_POINT ( 'NONE',  ( -5.923783695726434040, -7.499999999999999112, -16.97504159551249359 ) ) ;
#9714=ORIENTED_EDGE ( 'NONE', *, *, #14505, .T. ) ;
#9718=ORIENTED_EDGE ( 'NONE', *, *, #11215, .T. ) ;
#9722=DIRECTION ( 'NONE',  ( -1.000000000000000000, 0.000000000000000000, -0.000000000000000000 ) ) ;
#9727=CARTESIAN_POINT ( 'NONE',  ( 6.538348415311011408, 2.499999999999998224, -12.00000000000000000 ) ) ;
#9740=ADVANCED_FACE ( 'NONE', ( #8598 ), #6890, .T. ) ;
#9741=VERTEX_POINT ( 'NONE', #1149 ) ;
#9753=CARTESIAN_POINT ( 'NONE',  ( 0.000000000000000000, 0.000000000000000000, -3.000000000000000000 ) ) ;
#9771=CARTESIAN_POINT ( 'NONE',  ( 0.000000000000000000, 0.000000000000000000, -22.00000000000000000 ) ) ;
#9785=CARTESIAN_POINT ( 'NONE',  ( 0.000000000000000000, 0.000000000000000000, -12.00000000000000000 ) ) ;
#9817=VECTOR ( 'NONE', #5852, 1000.000000000000000 ) ;
#9862=EDGE_CURVE ( 'NONE', #6378, #622, #1039, .T. ) ;
#9863=EDGE_LOOP ( 'NONE', ( #11763, #1222, #18427, #16324, #6768, #14069 ) ) ;
#9864=FACE_OUTER_BOUND ( 'NONE', #14553, .T. ) ;
#9907=CARTESIAN_POINT ( 'NONE',  ( 1.089171355198147673, 7.499999999999999112, -14.58290923294918606 ) ) ;
#9917=CARTESIAN_POINT ( 'NONE',  ( 25.00000000000000000, -7.500000000000000888, -22.00000000000000000 ) ) ;
#9950=ORIENTED_EDGE ( 'NONE', *, *, #10896, .T. ) ;
#9963=ADVANCED_FACE ( 'NONE', ( #2616 ), #2346, .T. ) ;
#9981=DIRECTION ( 'NONE',  ( 0.000000000000000000, 0.000000000000000000, 1.000000000000000000 ) ) ;
#9995=DIRECTION ( 'NONE',  ( 0.000000000000000000, 1.000000000000000000, 0.000000000000000000 ) ) ;
#9997=CARTESIAN_POINT ( 'NONE',  ( -20.00000000000000000, -2.500000000000000444, -22.00000000000000000 ) ) ;
#10002=CARTESIAN_POINT ( 'NONE',  ( 2.482385025457376937, 7.499999999999866773, -13.17615586950464035 ) ) ;
#10017=ADVANCED_FACE ( 'NONE', ( #12846 ), #4162, .T. ) ;
#10033=DIRECTION ( 'NONE',  ( 1.335737076502141147E-14, 0.000000000000000000, -1.000000000000000000 ) ) ;
#10065=DIRECTION ( 'NONE',  ( 0.000000000000000000, -0.000000000000000000, 1.000000000000000000 ) ) ;
#10080=CIRCLE ( 'NONE', #13399, 7.000000000000000000 ) ;
#10092=CARTESIAN_POINT ( 'NONE',  ( -20.00000000000000000, 2.499999999999998668, -17.00000000000000000 ) ) ;
#10101=CARTESIAN_POINT ( 'NONE',  ( 0.9342146476565840185, 7.500000000000134115, -13.05973490260135073 ) ) ;
#10118=ORIENTED_EDGE ( 'NONE', *, *, #11526, .T. ) ;
#10163=EDGE_LOOP ( 'NONE', ( #13075, #11345, #14901, #2525 ) ) ;
#10178=AXIS2_PLACEMENT_3D ( 'NONE', #100, #8883, #10033 ) ;
#10182=AXIS2_PLACEMENT_3D ( 'NONE', #17975, #4877, #11175 ) ;
#10188=DIRECTION ( 'NONE',  ( 0.000000000000000000, -1.000000000000000000, 0.000000000000000000 ) ) ;
#10204=AXIS2_PLACEMENT_3D ( 'NONE', #4657, #15066, #4563 ) ;
#10213=AXIS2_PLACEMENT_3D ( 'NONE', #3322, #376, #13553 ) ;
#10220=CARTESIAN_POINT ( 'NONE',  ( -20.00000000000000000, -7.500000000000000888, -17.00000000000000000 ) ) ;
#10223=LINE ( 'NONE', #194, #18136 ) ;
#10229=PRODUCT_DEFINITION ( 'UNKNOWN', '', #8077, #7728 ) ;
#10241=CARTESIAN_POINT ( 'NONE',  ( 5.052632128771786135, -7.500000000000000888, -16.81774875490144794 ) ) ;
#10293=EDGE_CURVE ( 'NONE', #16711, #13920, #807, .T. ) ;
#10306=AXIS2_PLACEMENT_3D ( 'NONE', #2093, #18229, #3413 ) ;
#10337=CARTESIAN_POINT ( 'NONE',  ( 6.500524771653974021, -7.499999999999484857, -12.09892167832712850 ) ) ;
#10338=ORIENTED_EDGE ( 'NONE', *, *, #9424, .F. ) ;
#10367=CIRCLE ( 'NONE', #1514, 2.500000000000000000 ) ;
#10382=ORIENTED_EDGE ( 'NONE', *, *, #9599, .F. ) ;
#10410=CARTESIAN_POINT ( 'NONE',  ( -3.647233657245695149, 7.499999999999998224, -16.29053473562044019 ) ) ;
#10412=CARTESIAN_POINT ( 'NONE',  ( -6.538348415311011408, 7.500000000000000000, -12.00000000000000000 ) ) ;
#10424=EDGE_CURVE ( 'NONE', #12162, #17649, #10223, .T. ) ;
#10432=CARTESIAN_POINT ( 'NONE',  ( 4.545271119321602882, -5.336083332030053583, -11.99999999554311536 ) ) ;
#10475=AXIS2_PLACEMENT_3D ( 'NONE', #1195, #1096, #2519 ) ;
#10500=MANIFOLD_SOLID_BREP ( 'AdvancedHole1', #8171 ) ;
#10505=AXIS2_PLACEMENT_3D ( 'NONE', #17762, #17857, #3013 ) ;
#10506=CYLINDRICAL_SURFACE ( 'NONE', #2289, 5.000000000000000000 ) ;
#10511=CARTESIAN_POINT ( 'NONE',  ( 1.333872087798561257, 7.499999999999997335, -14.76174338479137838 ) ) ;
#10514=CARTESIAN_POINT ( 'NONE',  ( -25.00000000000000000, -2.500000000000000444, -17.00000000000000000 ) ) ;
#10529=CARTESIAN_POINT ( 'NONE',  ( 4.227723179940988452, -5.599337756632702501, -12.00000000790605093 ) ) ;
#10533=AXIS2_PLACEMENT_3D ( 'NONE', #94, #1329, #5908 ) ;
#10569=CARTESIAN_POINT ( 'NONE',  ( -20.00000000000000000, 2.499999999999998668, -16.99999999999999645 ) ) ;
#10608=EDGE_CURVE ( 'NONE', #9678, #4154, #13555, .T. ) ;
#10614=ORIENTED_EDGE ( 'NONE', *, *, #14024, .F. ) ;
#10625=DIRECTION ( 'NONE',  ( -1.000000000000000000, -0.000000000000000000, 0.000000000000000000 ) ) ;
#10633=CARTESIAN_POINT ( 'NONE',  ( -5.682963807814245705, -7.500000000000001776, -12.81889723681861248 ) ) ;
#10645=DIRECTION ( 'NONE',  ( 1.000000000000000000, 0.000000000000000000, 0.000000000000000000 ) ) ;
#10654=EDGE_CURVE ( 'NONE', #18897, #5701, #15989, .T. ) ;
#10656=ORIENTED_EDGE ( 'NONE', *, *, #16880, .F. ) ;
#10658=EDGE_LOOP ( 'NONE', ( #10382, #5946, #6675 ) ) ;
#10708=CARTESIAN_POINT ( 'NONE',  ( -5.084818453916207126, 7.500000000000262013, -13.03762002034318357 ) ) ;
#10723=CARTESIAN_POINT ( 'NONE',  ( -1.070106460717440422, -7.499999999999997335, -13.06798451319506249 ) ) ;
#10774=CARTESIAN_POINT ( 'NONE',  ( 2.863953186090933745, -7.500000000000002665, -15.84864299207353433 ) ) ;
#10777=ORIENTED_EDGE ( 'NONE', *, *, #8942, .T. ) ;
#10785=DIRECTION ( 'NONE',  ( 1.000000000000000000, 0.000000000000000000, 0.000000000000000000 ) ) ;
#10788=EDGE_LOOP ( 'NONE', ( #11592, #1296, #1929, #16733 ) ) ;
#10803=CARTESIAN_POINT ( 'NONE',  ( -6.265543861956235361, 7.499999999999998224, -12.41474642440600640 ) ) ;
#10805=DIRECTION ( 'NONE',  ( 0.000000000000000000, 0.000000000000000000, -1.000000000000000000 ) ) ;
#10817=CARTESIAN_POINT ( 'NONE',  ( 0.3417098569972104594, -7.500000000000000888, -14.22469181348825096 ) ) ;
#10821=DIRECTION ( 'NONE',  ( 1.000000000000000000, 0.000000000000000000, 0.000000000000000000 ) ) ;
#10846=ORIENTED_EDGE ( 'NONE', *, *, #14437, .T. ) ;
#10862=CIRCLE ( 'NONE', #14491, 5.000000000000000888 ) ;
#10878=CARTESIAN_POINT ( 'NONE',  ( -0.2640320147533066208, -7.500000000000001776, -14.20017596028259277 ) ) ;
#10884=LINE ( 'NONE', #833, #7582 ) ;
#10889=STYLED_ITEM ( 'NONE', ( #2066 ), #5561 ) ;
#10891=ORIENTED_EDGE ( 'NONE', *, *, #17354, .T. ) ;
#10896=EDGE_CURVE ( 'NONE', #8069, #16711, #1932, .T. ) ;
#10904=CARTESIAN_POINT ( 'NONE',  ( -1.149970134828562696, 6.907561563897650636, -11.99999999384793270 ) ) ;
#10920=CARTESIAN_POINT ( 'NONE',  ( -1.824285781648417037, -7.500000000000000888, -15.12168601478888874 ) ) ;
#10928=DIRECTION ( 'NONE',  ( 1.000000000000000000, 0.000000000000000000, 0.000000000000000000 ) ) ;
#10953=LINE ( 'NONE', #13892, #14118 ) ;
#10963=ORIENTED_EDGE ( 'NONE', *, *, #8485, .F. ) ;
#10968=CARTESIAN_POINT ( 'NONE',  ( 3.647233657245696925, -7.500000000000000888, -16.29053473562044019 ) ) ;
#10995=CARTESIAN_POINT ( 'NONE',  ( 0.5119965487701979567, 7.499999999999962697, -13.04039602617943672 ) ) ;
#10998=PRESENTATION_STYLE_ASSIGNMENT (( #2017 ) ) ;
#11009=CARTESIAN_POINT ( 'NONE',  ( -4.238775304281396927, -7.500000000000402345, -13.18441022661327011 ) ) ;
#11051=FACE_OUTER_BOUND ( 'NONE', #12249, .T. ) ;
#11057=CARTESIAN_POINT ( 'NONE',  ( -2.066926351139552143, -7.500000000000001776, -15.30321684074790234 ) ) ;
#11066=EDGE_CURVE ( 'NONE', #9395, #16458, #5768, .T. ) ;
#11069=ORIENTED_EDGE ( 'NONE', *, *, #2377, .F. ) ;
#11077=CARTESIAN_POINT ( 'NONE',  ( -20.00000000000000000, -2.500000000000000444, -17.00000000000000000 ) ) ;
#11084=CARTESIAN_POINT ( 'NONE',  ( 6.538348415311014072, -2.500000000000000444, -17.00000000000000000 ) ) ;
#11085=CARTESIAN_POINT ( 'NONE',  ( -2.048748540252033123, 6.701137625570393830, -11.99999999225504510 ) ) ;
#11100=CARTESIAN_POINT ( 'NONE',  ( -5.856338620593649402, -7.500000000000000000, -12.72522090842701736 ) ) ;
#11106=CARTESIAN_POINT ( 'NONE',  ( 20.00000000000000000, 0.000000000000000000, -22.00000000000000000 ) ) ;
#11124=EDGE_CURVE ( 'NONE', #11848, #16458, #9249, .T. ) ;
#11137=FACE_OUTER_BOUND ( 'NONE', #5617, .T. ) ;
#11175=DIRECTION ( 'NONE',  ( 1.000000000000000000, 0.000000000000000000, 0.000000000000000000 ) ) ;
#11176=CARTESIAN_POINT ( 'NONE',  ( 6.500003738483226989, 7.499999999998957279, -12.10028435765586252 ) ) ;
#11179=CARTESIAN_POINT ( 'NONE',  ( 0.000000000000000000, 0.000000000000000000, -12.00000000000000000 ) ) ;
#11184=LINE ( 'NONE', #5246, #9104 ) ;
#11213=AXIS2_PLACEMENT_3D ( 'NONE', #9785, #2515, #17060 ) ;
#11215=EDGE_CURVE ( 'NONE', #2949, #7506, #10953, .T. ) ;
#11237=CARTESIAN_POINT ( 'NONE',  ( 0.000000000000000000, 0.000000000000000000, 0.000000000000000000 ) ) ;
#11248=DIRECTION ( 'NONE',  ( 0.000000000000000000, 0.000000000000000000, 1.000000000000000000 ) ) ;
#11270=CARTESIAN_POINT ( 'NONE',  ( 6.273991221456205913, 3.109390318170344614, -12.00000000063437433 ) ) ;
#11276=DIRECTION ( 'NONE',  ( -0.000000000000000000, -0.000000000000000000, 1.000000000000000000 ) ) ;
#11287=CARTESIAN_POINT ( 'NONE',  ( -5.926008024970758292, -7.500000000000000888, -16.97528233579634716 ) ) ;
#11300=ORIENTED_EDGE ( 'NONE', *, *, #2048, .T. ) ;
#11325=DIRECTION ( 'NONE',  ( 1.000000000000000000, 0.000000000000000000, -0.000000000000000000 ) ) ;
#11345=ORIENTED_EDGE ( 'NONE', *, *, #10293, .T. ) ;
#11351=DIRECTION ( 'NONE',  ( 1.000000000000000000, 0.000000000000000000, 0.000000000000000000 ) ) ;
#11374=CARTESIAN_POINT ( 'NONE',  ( -5.324905852942846352, -7.500000000000000888, -16.88120503408574180 ) ) ;
#11390=VECTOR ( 'NONE', #13138, 1000.000000000000000 ) ;
#11399=DIRECTION ( 'NONE',  ( 1.000000000000000000, 0.000000000000000000, 0.000000000000000000 ) ) ;
#11404=ORIENTED_EDGE ( 'NONE', *, *, #7230, .F. ) ;
#11447=CARTESIAN_POINT ( 'NONE',  ( 3.338474662712863417, 7.499999999999999112, -16.12819240262157194 ) ) ;
#11449=CARTESIAN_POINT ( 'NONE',  ( 25.00000000000000000, -2.500000000000000444, -12.00000000000000000 ) ) ;
#11469=LINE ( 'NONE', #14514, #5951 ) ;
#11473=VECTOR ( 'NONE', #8323, 1000.000000000000000 ) ;
#11477=DIRECTION ( 'NONE',  ( 0.000000000000000000, -1.000000000000000000, 0.000000000000000000 ) ) ;
#11526=EDGE_CURVE ( 'NONE', #4766, #16711, #7131, .T. ) ;
#11543=CARTESIAN_POINT ( 'NONE',  ( 5.250594443112312604, 4.638468187398189002, -11.99999999738841083 ) ) ;
#11563=EDGE_LOOP ( 'NONE', ( #7042, #2980, #10846, #7932, #18051 ) ) ;
#11566=DIRECTION ( 'NONE',  ( -1.000000000000000000, 0.000000000000000000, 0.000000000000000000 ) ) ;
#11585=CARTESIAN_POINT ( 'NONE',  ( 2.864513242452144226, -7.500000000000000888, -15.84899838955148432 ) ) ;
#11587=DIRECTION ( 'NONE',  ( 1.000000000000000000, 0.000000000000000000, 0.000000000000000000 ) ) ;
#11592=ORIENTED_EDGE ( 'NONE', *, *, #15896, .T. ) ;
#11597=LINE ( 'NONE', #2871, #3706 ) ;
#11608=DIRECTION ( 'NONE',  ( -6.938893903907227392E-16, 0.000000000000000000, 1.000000000000000000 ) ) ;
#11668=ORIENTED_EDGE ( 'NONE', *, *, #8176, .T. ) ;
#11673=CARTESIAN_POINT ( 'NONE',  ( 5.288115175735552675, -4.595214139558242650, -11.99999999743901746 ) ) ;
#11674=SHAPE_REPRESENTATION ( 'Ergonomic Rotary Turning Knob', ( #2030 ), #9034 ) ;
#11677=DIRECTION ( 'NONE',  ( -0.8571673007021134438, 1.049727191138620051E-16, 0.5150380749100522682 ) ) ;
#11679=FACE_OUTER_BOUND ( 'NONE', #8917, .T. ) ;
#11686=CARTESIAN_POINT ( 'NONE',  ( 0.000000000000000000, 0.000000000000000000, -12.00000000000000000 ) ) ;
#11690=EDGE_CURVE ( 'NONE', #4766, #8069, #8954, .T. ) ;
#11696=ORIENTED_EDGE ( 'NONE', *, *, #11755, .T. ) ;
#11723=CARTESIAN_POINT ( 'NONE',  ( 20.00000000000000000, -2.500000000000000444, -16.99999999999999645 ) ) ;
#11754=CARTESIAN_POINT ( 'NONE',  ( -6.500132120881464637, 2.599948583552246451, -12.00000000000000000 ) ) ;
#11755=EDGE_CURVE ( 'NONE', #13344, #4154, #1627, .T. ) ;
#11759=AXIS2_PLACEMENT_3D ( 'NONE', #7729, #13538, #7827 ) ;
#11763=ORIENTED_EDGE ( 'NONE', *, *, #16473, .T. ) ;
#11773=CARTESIAN_POINT ( 'NONE',  ( 6.454593536054717973, -2.712332671582271093, -12.00000000018537882 ) ) ;
#11793=EDGE_LOOP ( 'NONE', ( #7795, #13409, #8754, #13611 ) ) ;
#11848=VERTEX_POINT ( 'NONE', #14339 ) ;
#11849=CARTESIAN_POINT ( 'NONE',  ( -1.391363329066502619, 7.500000000000000000, -14.80343650618309326 ) ) ;
#11850=CIRCLE ( 'NONE', #16447, 7.000000000000000000 ) ;
#11851=SPHERICAL_SURFACE ( 'NONE', #8968, 5.000000000000000000 ) ;
#11852=DIRECTION ( 'NONE',  ( 0.000000000000000000, 1.000000000000000000, 0.000000000000000000 ) ) ;
#11868=CARTESIAN_POINT ( 'NONE',  ( 3.648056509801858027, -7.500000000000000888, -16.29094785500087994 ) ) ;
#11875=ADVANCED_FACE ( 'NONE', ( #16054 ), #2948, .T. ) ;
#11907=DIRECTION ( 'NONE',  ( -0.000000000000000000, -0.000000000000000000, 1.000000000000000000 ) ) ;
#11918=ORIENTED_EDGE ( 'NONE', *, *, #14975, .F. ) ;
#11934=FACE_OUTER_BOUND ( 'NONE', #4429, .T. ) ;
#11946=CARTESIAN_POINT ( 'NONE',  ( -6.538348415311010520, -2.500000000000000444, -12.00000000000000000 ) ) ;
#11947=DIRECTION ( 'NONE',  ( 0.000000000000000000, 0.000000000000000000, -1.000000000000000000 ) ) ;
#11957=ORIENTED_EDGE ( 'NONE', *, *, #2325, .T. ) ;
#11963=CARTESIAN_POINT ( 'NONE',  ( 2.953963787679646735, -6.378445150919258566, -12.00000001548996487 ) ) ;
#11986=ORIENTED_EDGE ( 'NONE', *, *, #16857, .T. ) ;
#11999=( NAMED_UNIT ( * ) SI_UNIT ( $, .STERADIAN. ) SOLID_ANGLE_UNIT ( ) );
#12002=CARTESIAN_POINT ( 'NONE',  ( 6.538348415311010520, 7.499999999999999112, -16.99999999999999645 ) ) ;
#12005=CARTESIAN_POINT ( 'NONE',  ( -25.00000000000000000, 2.499999999999998668, -17.00000000000000000 ) ) ;
#12042=CARTESIAN_POINT ( 'NONE',  ( -4.478293880065214339, 7.500000000000000888, -16.64373187125687181 ) ) ;
#12061=CARTESIAN_POINT ( 'NONE',  ( -1.454043889487635077, -7.499999999999869438, -13.09460583645939558 ) ) ;
#12076=DIRECTION ( 'NONE',  ( -0.000000000000000000, -0.000000000000000000, 1.000000000000000000 ) ) ;
#12084=EDGE_LOOP ( 'NONE', ( #16869, #393, #6606 ) ) ;
#12085=EDGE_LOOP ( 'NONE', ( #16789, #837, #10614 ) ) ;
#12096=COLOUR_RGB ( '', 0.66274510, 0.83137255, 0.94901961) ;
#12118=CIRCLE ( 'NONE', #6005, 5.000000000000000888 ) ;
#12138=SPHERICAL_SURFACE ( 'NONE', #10213, 5.000000000000000000 ) ;
#12143=CARTESIAN_POINT ( 'NONE',  ( 5.027901255400304414, 7.499999999999997335, -16.81159201184367902 ) ) ;
#12146=CARTESIAN_POINT ( 'NONE',  ( -4.479409541426045749, 7.499999999999999112, -16.64412940056556067 ) ) ;
#12161=CARTESIAN_POINT ( 'NONE',  ( 0.1174197124922954222, -7.500000000000000888, -14.18273494860523520 ) ) ;
#12162=VERTEX_POINT ( 'NONE', #12002 ) ;
#12170=CARTESIAN_POINT ( 'NONE',  ( 20.00000000000000000, 2.499999999999998668, -17.00000000000000000 ) ) ;
#12211=DIRECTION ( 'NONE',  ( -1.000000000000000000, 6.938893903907227392E-16, 0.000000000000000000 ) ) ;
#12224=EDGE_LOOP ( 'NONE', ( #5348, #3269, #17040, #14105 ) ) ;
#12235=CARTESIAN_POINT ( 'NONE',  ( -1.149044392847440088, 7.500000000000000000, -14.62466132081332582 ) ) ;
#12239=CARTESIAN_POINT ( 'NONE',  ( -0.9490252293515478721, 6.938433416811056631, -12.00000000290481239 ) ) ;
#12243=FACE_OUTER_BOUND ( 'NONE', #18101, .T. ) ;
#12249=EDGE_LOOP ( 'NONE', ( #15824, #2026, #4821 ) ) ;
#12251=CARTESIAN_POINT ( 'NONE',  ( -0.3159797039860490209, -6.996005774985150083, -11.99999999647927496 ) ) ;
#12287=SPHERICAL_SURFACE ( 'NONE', #17619, 5.000000000000000000 ) ;
#12299=ORIENTED_EDGE ( 'NONE', *, *, #18832, .F. ) ;
#12300=DIRECTION ( 'NONE',  ( 1.000000000000000000, -0.000000000000000000, -0.000000000000000000 ) ) ;
#12307=ORIENTED_EDGE ( 'NONE', *, *, #5123, .F. ) ;
#12323=CARTESIAN_POINT ( 'NONE',  ( 0.3159797039863193602, 6.996005774985157188, -11.99999999647930871 ) ) ;
#12328=DIRECTION ( 'NONE',  ( 1.000000000000000000, 0.000000000000000000, 0.000000000000000000 ) ) ;
#12335=CARTESIAN_POINT ( 'NONE',  ( -0.5544330523543454792, -7.500000000000000888, -14.29923508549715194 ) ) ;
#12338=LINE ( 'NONE', #6612, #16706 ) ;
#12342=EDGE_CURVE ( 'NONE', #622, #16531, #8441, .T. ) ;
#12353=CARTESIAN_POINT ( 'NONE',  ( -25.00000000000000000, -7.500000000000000888, -17.00000000000000000 ) ) ;
#12370=PRODUCT_CONTEXT ( 'NONE', #12539, 'mechanical' ) ;
#12396=ORIENTED_EDGE ( 'NONE', *, *, #11690, .T. ) ;
#12401=VERTEX_POINT ( 'NONE', #15889 ) ;
#12411=CARTESIAN_POINT ( 'NONE',  ( 6.538348415311010520, 7.499999999999999112, -16.99999999999999645 ) ) ;
#12413=AXIS2_PLACEMENT_3D ( 'NONE', #394, #14914, #1930 ) ;
#12416=CARTESIAN_POINT ( 'NONE',  ( 0.7340363079801778268, 6.964562493341673211, -12.00000000352069307 ) ) ;
#12433=CARTESIAN_POINT ( 'NONE',  ( -5.763005853485871910, -3.979914285031270538, -11.99999999870361655 ) ) ;
#12438=DIRECTION ( 'NONE',  ( 0.000000000000000000, -0.000000000000000000, -1.000000000000000000 ) ) ;
#12468=PLANE ( 'NONE',  #6336 ) ;
#12471=EDGE_CURVE ( 'NONE', #18780, #8559, #11597, .T. ) ;
#12477=CARTESIAN_POINT ( 'NONE',  ( 6.236214402462485040, -7.500000000000000000, -16.99999999999999645 ) ) ;
#12483=AXIS2_PLACEMENT_3D ( 'NONE', #18354, #2389, #10821 ) ;
#12502=CARTESIAN_POINT ( 'NONE',  ( -0.7622588538374093226, 7.499999999999999112, -14.39637362139732346 ) ) ;
#12538=EDGE_CURVE ( 'NONE', #18705, #5896, #15128, .T. ) ;
#12539=APPLICATION_CONTEXT ( 'automotive_design' ) ;
#12566=CARTESIAN_POINT ( 'NONE',  ( -0.6933513387705726450, -7.500000000000003553, -14.36029122898769117 ) ) ;
#12567=CARTESIAN_POINT ( 'NONE',  ( 25.00000000000000000, 7.499999999999999112, -22.00000000000000000 ) ) ;
#12586=CARTESIAN_POINT ( 'NONE',  ( 5.923783695726432263, 7.500000000000000000, -16.97504159551249359 ) ) ;
#12589=CARTESIAN_POINT ( 'NONE',  ( 6.437519407326084853, 7.499999999999865885, -12.20843479742065441 ) ) ;
#12602=AXIS2_PLACEMENT_3D ( 'NONE', #12170, #17999, #316 ) ;
#12649=DIRECTION ( 'NONE',  ( 0.000000000000000000, 0.000000000000000000, -1.000000000000000000 ) ) ;
#12655=AXIS2_PLACEMENT_3D ( 'NONE', #1299, #18596, #9995 ) ;
#12658=FACE_OUTER_BOUND ( 'NONE', #11563, .T. ) ;
#12686=CARTESIAN_POINT ( 'NONE',  ( 5.763005853485449137, 3.979914285031491694, -11.99999999870348688 ) ) ;
#12703=CARTESIAN_POINT ( 'NONE',  ( -6.437519407326167453, -7.499999999999735323, -12.20843479742017657 ) ) ;
#12724=AXIS2_PLACEMENT_3D ( 'NONE', #1350, #7195, #11587 ) ;
#12737=ORIENTED_EDGE ( 'NONE', *, *, #8215, .T. ) ;
#12743=FACE_OUTER_BOUND ( 'NONE', #17770, .T. ) ;
#12766=VERTEX_POINT ( 'NONE', #2760 ) ;
#12778=CARTESIAN_POINT ( 'NONE',  ( 3.324307330593150756, 6.179741886604479539, -11.99999999169344633 ) ) ;
#12803=CARTESIAN_POINT ( 'NONE',  ( 0.000000000000000000, 0.000000000000000000, 0.000000000000000000 ) ) ;
#12810=CARTESIAN_POINT ( 'NONE',  ( 20.00000000000000000, -2.500000000000000444, -16.99999999999999645 ) ) ;
#12821=CARTESIAN_POINT ( 'NONE',  ( 0.000000000000000000, 0.000000000000000000, -3.000000000000000000 ) ) ;
#12846=FACE_OUTER_BOUND ( 'NONE', #9863, .T. ) ;
#12867=CARTESIAN_POINT ( 'NONE',  ( 2.826946895708269736, 6.438259034076401655, -12.00000001686870732 ) ) ;
#12942=PLANE ( 'NONE',  #15120 ) ;
#12953=VECTOR ( 'NONE', #1689, 1000.000000000000000 ) ;
#12959=CARTESIAN_POINT ( 'NONE',  ( 25.00000000000000000, 2.499999999999998668, -17.00000000000000000 ) ) ;
#12962=CARTESIAN_POINT ( 'NONE',  ( 5.682963807814618740, 7.499999999999998224, -12.81889723681830695 ) ) ;
#13036=DIRECTION ( 'NONE',  ( -1.000000000000000000, 0.000000000000000000, -6.938893903907225419E-16 ) ) ;
#13075=ORIENTED_EDGE ( 'NONE', *, *, #1831, .F. ) ;
#13129=CARTESIAN_POINT ( 'NONE',  ( 2.179449471770337432, -4.500000000000000000, 0.000000000000000000 ) ) ;
#13138=DIRECTION ( 'NONE',  ( 0.000000000000000000, 0.000000000000000000, 1.000000000000000000 ) ) ;
#13178=PLANE ( 'NONE',  #10533 ) ;
#13181=FACE_OUTER_BOUND ( 'NONE', #6852, .T. ) ;
#13200=CARTESIAN_POINT ( 'NONE',  ( -5.000000000000000000, 6.123233995736766282E-16, 0.000000000000000000 ) ) ;
#13280=AXIS2_PLACEMENT_3D ( 'NONE', #7460, #186, #14608 ) ;
#13290=ADVANCED_FACE ( 'NONE', ( #12243 ), #8221, .T. ) ;
#13293=CARTESIAN_POINT ( 'NONE',  ( 5.308815406012384663, -7.500000000000255795, -12.96907596528278184 ) ) ;
#13316=VERTEX_POINT ( 'NONE', #4972 ) ;
#13324=PRODUCT_DEFINITION_SHAPE ( 'NONE', 'NONE',  #10229 ) ;
#13332=AXIS2_PLACEMENT_3D ( 'NONE', #1698, #467, #7545 ) ;
#13335=AXIS2_PLACEMENT_3D ( 'NONE', #229, #9016, #17816 ) ;
#13344=VERTEX_POINT ( 'NONE', #8394 ) ;
#13346=AXIS2_PLACEMENT_3D ( 'NONE', #4551, #11907, #16310 ) ;
#13365=ORIENTED_EDGE ( 'NONE', *, *, #13633, .F. ) ;
#13367=ORIENTED_EDGE ( 'NONE', *, *, #1315, .F. ) ;
#13373=CARTESIAN_POINT ( 'NONE',  ( 1.088636994872527408, 7.500000000000000000, -14.58255216580684177 ) ) ;
#13385=EDGE_LOOP ( 'NONE', ( #16945, #6194, #7693, #10656 ) ) ;
#13391=CARTESIAN_POINT ( 'NONE',  ( 6.500132120881376707, -2.599948583552213144, -12.00000000000000000 ) ) ;
#13399=AXIS2_PLACEMENT_3D ( 'NONE', #7077, #3924, #11566 ) ;
#13409=ORIENTED_EDGE ( 'NONE', *, *, #18195, .T. ) ;
#13413=EDGE_LOOP ( 'NONE', ( #4978, #4332, #15827 ) ) ;
#13430=DIRECTION ( 'NONE',  ( 0.000000000000000000, -0.000000000000000000, 1.000000000000000000 ) ) ;
#13440=AXIS2_PLACEMENT_3D ( 'NONE', #17314, #2861, #17 ) ;
#13483=CARTESIAN_POINT ( 'NONE',  ( 4.294575106067288317, -7.500000000000266454, -13.17881115347054788 ) ) ;
#13535=FACE_OUTER_BOUND ( 'NONE', #5752, .T. ) ;
#13538=DIRECTION ( 'NONE',  ( 0.000000000000000000, 0.000000000000000000, -1.000000000000000000 ) ) ;
#13546=FACE_OUTER_BOUND ( 'NONE', #10788, .T. ) ;
#13553=DIRECTION ( 'NONE',  ( -1.000000000000000000, 6.938893903907227392E-16, 0.000000000000000000 ) ) ;
#13555=CIRCLE ( 'NONE', #5309, 7.000000000000000000 ) ;
#13560=ORIENTED_EDGE ( 'NONE', *, *, #15488, .T. ) ;
#13561=CARTESIAN_POINT ( 'NONE',  ( 5.322906077793303048, 7.499999999999998224, -16.88078391064166084 ) ) ;
#13581=CARTESIAN_POINT ( 'NONE',  ( -0.2633197948916921605, -7.500000000000000888, -14.20553286501775858 ) ) ;
#13589=AXIS2_PLACEMENT_3D ( 'NONE', #10092, #15922, #17653 ) ;
#13610=ADVANCED_FACE ( 'NONE', ( #8106 ), #16727, .F. ) ;
#13611=ORIENTED_EDGE ( 'NONE', *, *, #15246, .F. ) ;
#13616=EDGE_CURVE ( 'NONE', #13920, #5818, #5426, .T. ) ;
#13633=EDGE_CURVE ( 'NONE', #17649, #18897, #10884, .T. ) ;
#13670=CARTESIAN_POINT ( 'NONE',  ( -1.715145640899952140, 6.797472175340259604, -12.00000001230413460 ) ) ;
#13682=ORIENTED_EDGE ( 'NONE', *, *, #17218, .T. ) ;
#13684=CARTESIAN_POINT ( 'NONE',  ( -0.09864563712516453975, -7.002566078024231366, -11.99999999788115446 ) ) ;
#13733=CARTESIAN_POINT ( 'NONE',  ( 1.149044392847440088, -7.500000000000001776, -14.62466132081333292 ) ) ;
#13747=CARTESIAN_POINT ( 'NONE',  ( 2.179449471770337432, -4.500000000000000000, -3.000000000000000000 ) ) ;
#13756=CARTESIAN_POINT ( 'NONE',  ( -0.1927609796802092212, 7.499999999999999112, -14.19253746125318116 ) ) ;
#13772=CARTESIAN_POINT ( 'NONE',  ( 0.6634400264851448847, -7.500000000000235367, -13.04619536630284493 ) ) ;
#13782=CARTESIAN_POINT ( 'NONE',  ( -2.500000000000000000, 3.061616997868383141E-16, -3.000000000000000000 ) ) ;
#13796=AXIS2_PLACEMENT_3D ( 'NONE', #13747, #659, #3615 ) ;
#13843=CARTESIAN_POINT ( 'NONE',  ( -0.8060261380169082557, 7.500000000000031086, -13.05296413415600298 ) ) ;
#13853=CIRCLE ( 'NONE', #3156, 5.000000000000000888 ) ;
#13859=CARTESIAN_POINT ( 'NONE',  ( -0.03525595549294711917, -7.500000000000000888, -14.17755750872192522 ) ) ;
#13865=AXIS2_PLACEMENT_3D ( 'NONE', #1646, #12076, #10645 ) ;
#13886=FACE_OUTER_BOUND ( 'NONE', #8789, .T. ) ;
#13892=CARTESIAN_POINT ( 'NONE',  ( 2.500000000000000000, 0.000000000000000000, -13.00000000000000533 ) ) ;
#13909=CARTESIAN_POINT ( 'NONE',  ( 5.342326914280424610, -7.500000000000001776, -16.88455910646441538 ) ) ;
#13911=CARTESIAN_POINT ( 'NONE',  ( -20.00000000000000000, -2.500000000000000444, -17.00000000000000000 ) ) ;
#13920=VERTEX_POINT ( 'NONE', #6075 ) ;
#13923=ORIENTED_EDGE ( 'NONE', *, *, #2463, .F. ) ;
#13934=CIRCLE ( 'NONE', #13335, 7.000000000000000000 ) ;
#13936=CARTESIAN_POINT ( 'NONE',  ( -2.166051897649948543, 7.500000000000000000, -13.14980647003224767 ) ) ;
#13946=AXIS2_PLACEMENT_3D ( 'NONE', #9753, #17395, #968 ) ;
#13951=AXIS2_PLACEMENT_3D ( 'NONE', #6963, #5503, #11351 ) ;
#14001=EDGE_LOOP ( 'NONE', ( #14031, #1856, #9418, #11069 ) ) ;
#14007=CARTESIAN_POINT ( 'NONE',  ( -3.605312816022526956, -7.500000000000002665, -16.26975837274199677 ) ) ;
#14010=CARTESIAN_POINT ( 'NONE',  ( 20.00000000000000000, 7.499999999999999112, -12.00000000000000000 ) ) ;
#14024=EDGE_CURVE ( 'NONE', #5848, #5701, #9701, .T. ) ;
#14031=ORIENTED_EDGE ( 'NONE', *, *, #4337, .T. ) ;
#14034=CARTESIAN_POINT ( 'NONE',  ( -5.343731732829805736, 7.499999999999999112, -16.88485148858611140 ) ) ;
#14052=CARTESIAN_POINT ( 'NONE',  ( 2.500000000000000000, 0.000000000000000000, -13.00000000000000533 ) ) ;
#14055=FACE_OUTER_BOUND ( 'NONE', #9619, .T. ) ;
#14069=ORIENTED_EDGE ( 'NONE', *, *, #5290, .T. ) ;
#14076=AXIS2_PLACEMENT_3D ( 'NONE', #5151, #16815, #9547 ) ;
#14083=PLANE ( 'NONE',  #569 ) ;
#14103=ADVANCED_FACE ( 'NONE', ( #2418 ), #14083, .F. ) ;
#14105=ORIENTED_EDGE ( 'NONE', *, *, #5123, .T. ) ;
#14116=CARTESIAN_POINT ( 'NONE',  ( 6.538348415311014072, 7.499999999999999112, -17.00000000000000000 ) ) ;
#14118=VECTOR ( 'NONE', #3383, 1000.000000000000000 ) ;
#14137=DIRECTION ( 'NONE',  ( -0.000000000000000000, 1.000000000000000000, 1.734723475976806848E-16 ) ) ;
#14175=AXIS2_PLACEMENT_3D ( 'NONE', #8460, #2794, #15710 ) ;
#14194=CIRCLE ( 'NONE', #13589, 5.000000000000000000 ) ;
#14207=ORIENTED_EDGE ( 'NONE', *, *, #10424, .F. ) ;
#14215=FACE_OUTER_BOUND ( 'NONE', #3074, .T. ) ;
#14220=CARTESIAN_POINT ( 'NONE',  ( 1.824285781649040761, 7.499999999999999112, -15.12168601478843044 ) ) ;
#14225=AXIS2_PLACEMENT_3D ( 'NONE', #18487, #3965, #8188 ) ;
#14246=CARTESIAN_POINT ( 'NONE',  ( -20.00000000000000000, 0.000000000000000000, -16.99999999999999645 ) ) ;
#14247=CARTESIAN_POINT ( 'NONE',  ( -2.500000000000000000, 3.061616997868383141E-16, -3.000000000000000000 ) ) ;
#14283=VERTEX_POINT ( 'NONE', #1462 ) ;
#14313=CARTESIAN_POINT ( 'NONE',  ( 2.061733300930400858, 7.499999999999732658, -13.14107379030440370 ) ) ;
#14339=CARTESIAN_POINT ( 'NONE',  ( -5.000000000000000000, 6.123233995736766282E-16, 0.000000000000000000 ) ) ;
#14362=EDGE_CURVE ( 'NONE', #13344, #3494, #11184, .T. ) ;
#14392=FACE_OUTER_BOUND ( 'NONE', #16184, .T. ) ;
#14397=CARTESIAN_POINT ( 'NONE',  ( 4.525831033741626541, 7.500000000000000000, -13.14978481913310304 ) ) ;
#14398=DIRECTION ( 'NONE',  ( -0.000000000000000000, -0.000000000000000000, 1.000000000000000000 ) ) ;
#14413=DIRECTION ( 'NONE',  ( 1.000000000000000000, 0.000000000000000000, 0.000000000000000000 ) ) ;
#14422=DIRECTION ( 'NONE',  ( 0.000000000000000000, 1.000000000000000000, 0.000000000000000000 ) ) ;
#14437=EDGE_CURVE ( 'NONE', #322, #9741, #11850, .T. ) ;
#14443=CYLINDRICAL_SURFACE ( 'NONE', #12724, 2.500000000000000000 ) ;
#14467=CARTESIAN_POINT ( 'NONE',  ( 6.538348415311010520, 2.499999999999998668, -17.00000000000000000 ) ) ;
#14491=AXIS2_PLACEMENT_3D ( 'NONE', #11723, #10188, #7531 ) ;
#14505=EDGE_CURVE ( 'NONE', #1807, #14283, #15644, .T. ) ;
#14514=CARTESIAN_POINT ( 'NONE',  ( 7.000000000000000000, 0.000000000000000000, -12.00000000000000000 ) ) ;
#14535=CARTESIAN_POINT ( 'NONE',  ( 1.391479049022300574, -7.500000000000000888, -14.80352021213832536 ) ) ;
#14549=DIRECTION ( 'NONE',  ( -1.000000000000000000, 0.000000000000000000, 0.000000000000000000 ) ) ;
#14553=EDGE_LOOP ( 'NONE', ( #13682, #12737, #7264, #1785, #17274 ) ) ;
#14594=DIRECTION ( 'NONE',  ( -0.000000000000000000, 1.000000000000000000, 0.000000000000000000 ) ) ;
#14608=DIRECTION ( 'NONE',  ( -1.000000000000000000, 0.000000000000000000, 0.000000000000000000 ) ) ;
#14616=DIRECTION ( 'NONE',  ( 0.000000000000000000, 0.000000000000000000, -1.000000000000000000 ) ) ;
#14618=AXIS2_PLACEMENT_3D ( 'NONE', #14706, #8793, #17782 ) ;
#14620=VECTOR ( 'NONE', #11677, 1000.000000000000000 ) ;
#14623=ADVANCED_FACE ( 'NONE', ( #3112 ), #16031, .T. ) ;
#14625=ADVANCED_FACE ( 'NONE', ( #13546 ), #14788, .T. ) ;
#14632=EDGE_LOOP ( 'NONE', ( #197, #3753, #7696 ) ) ;
#14634=CARTESIAN_POINT ( 'NONE',  ( 2.611994420159011732, -7.500000000000000888, -15.68429332095010231 ) ) ;
#14650=ORIENTED_EDGE ( 'NONE', *, *, #13633, .T. ) ;
#14704=CARTESIAN_POINT ( 'NONE',  ( -0.7623231285407784386, 7.500000000000000000, -14.39641017501654829 ) ) ;
#14706=CARTESIAN_POINT ( 'NONE',  ( 0.000000000000000000, 0.000000000000000000, 0.000000000000000000 ) ) ;
#14723=CARTESIAN_POINT ( 'NONE',  ( 6.154177238273381256, -7.500000000000001776, -12.51861270110025792 ) ) ;
#14761=LINE ( 'NONE', #4450, #3569 ) ;
#14788=CYLINDRICAL_SURFACE ( 'NONE', #13332, 5.000000000000000888 ) ;
#14806=CARTESIAN_POINT ( 'NONE',  ( -6.454593536054757941, 2.712332671582286192, -12.00000000018538415 ) ) ;
#14824=CARTESIAN_POINT ( 'NONE',  ( 6.238556470687417921, -7.500000000000000888, -16.99999999974153297 ) ) ;
#14851=CIRCLE ( 'NONE', #12413, 5.000000000000000888 ) ;
#14896=FACE_OUTER_BOUND ( 'NONE', #4918, .T. ) ;
#14901=ORIENTED_EDGE ( 'NONE', *, *, #8046, .F. ) ;
#14902=CARTESIAN_POINT ( 'NONE',  ( 3.605312816022526512, 7.499999999999999112, -16.26975837274198966 ) ) ;
#14914=DIRECTION ( 'NONE',  ( -1.000000000000000000, -0.000000000000000000, 0.000000000000000000 ) ) ;
#14919=CARTESIAN_POINT ( 'NONE',  ( 5.935721797378563203, -7.500000000000000888, -16.97606798286663476 ) ) ;
#14932=CARTESIAN_POINT ( 'NONE',  ( 2.179449471770337432, -4.500000000000000000, -3.000000000000000000 ) ) ;
#14936=CIRCLE ( 'NONE', #5765, 5.000000000000000888 ) ;
#14975=EDGE_CURVE ( 'NONE', #8559, #5701, #14761, .T. ) ;
#15014=CARTESIAN_POINT ( 'NONE',  ( 0.3286731010499749361, -6.995544057484789136, -12.00000000211884554 ) ) ;
#15035=ORIENTED_EDGE ( 'NONE', *, *, #3240, .F. ) ;
#15053=CARTESIAN_POINT ( 'NONE',  ( 2.500000000000000000, 0.000000000000000000, -3.000000000000000000 ) ) ;
#15066=DIRECTION ( 'NONE',  ( -0.000000000000000000, 0.000000000000000000, 1.000000000000000000 ) ) ;
#15074=CIRCLE ( 'NONE', #5005, 5.000000000000000888 ) ;
#15077=VERTEX_POINT ( 'NONE', #15053 ) ;
#15094=CARTESIAN_POINT ( 'NONE',  ( -6.236214402462488593, 7.499999999999999112, -17.00000000000000355 ) ) ;
#15096=CARTESIAN_POINT ( 'NONE',  ( -1.391479049022228187, 7.499999999999999112, -14.80352021213800917 ) ) ;
#15113=CARTESIAN_POINT ( 'NONE',  ( -4.153045036173530491, -5.656186534233802021, -12.00000000830646840 ) ) ;
#15120=AXIS2_PLACEMENT_3D ( 'NONE', #12567, #4161, #16973 ) ;
#15128=LINE ( 'NONE', #14932, #7999 ) ;
#15132=VECTOR ( 'NONE', #11477, 1000.000000000000000 ) ;
#15135=CARTESIAN_POINT ( 'NONE',  ( 5.000000000000000000, 0.000000000000000000, 0.000000000000000000 ) ) ;
#15157=CARTESIAN_POINT ( 'NONE',  ( 20.00000000000000000, -2.500000000000000444, -12.00000000000000000 ) ) ;
#15171=LINE ( 'NONE', #16876, #16777 ) ;
#15175=CARTESIAN_POINT ( 'NONE',  ( 20.00000000000000000, -7.500000000000000888, -16.99999999999999645 ) ) ;
#15197=CARTESIAN_POINT ( 'NONE',  ( -0.1174197124920530882, 7.499999999999999112, -14.18273494860542705 ) ) ;
#15200=CARTESIAN_POINT ( 'NONE',  ( 20.00000000000000000, 0.000000000000000000, -16.99999999999999645 ) ) ;
#15212=CARTESIAN_POINT ( 'NONE',  ( -2.037104019874120375, -6.699095661347423736, -11.99999999578283294 ) ) ;
#15229=CARTESIAN_POINT ( 'NONE',  ( -20.00000000000000000, -2.500000000000000444, -12.00000000000000000 ) ) ;
#15241=SURFACE_STYLE_FILL_AREA ( #18202 ) ;
#15246=EDGE_CURVE ( 'NONE', #7506, #15077, #5294, .T. ) ;
#15258=CARTESIAN_POINT ( 'NONE',  ( 0.3448739086965406653, -7.500000000000000888, -14.22069309503974921 ) ) ;
#15283=CARTESIAN_POINT ( 'NONE',  ( -3.669726844813804956, 7.500000000000255795, -13.21471411064774237 ) ) ;
#15296=CARTESIAN_POINT ( 'NONE',  ( -5.616333669597630696, -4.188188789804105916, -12.00000000261157496 ) ) ;
#15299=ADVANCED_FACE ( 'NONE', ( #12743 ), #5557, .T. ) ;
#15341=PLANE ( 'NONE',  #14225 ) ;
#15342=CARTESIAN_POINT ( 'NONE',  ( 2.117556820461448996, -7.500000000000002665, -15.34001259936770722 ) ) ;
#15349=CARTESIAN_POINT ( 'NONE',  ( 0.000000000000000000, 0.000000000000000000, -13.00000000000000533 ) ) ;
#15370=CARTESIAN_POINT ( 'NONE',  ( -3.431439422792162741, 6.119758975833253345, -11.99999999209397572 ) ) ;
#15389=CARTESIAN_POINT ( 'NONE',  ( -4.525831033740718823, -7.499999999999870326, -13.14978481913338371 ) ) ;
#15407=AXIS2_PLACEMENT_3D ( 'NONE', #643, #558, #12211 ) ;
#15418=DIRECTION ( 'NONE',  ( 1.000000000000000000, 0.000000000000000000, 0.000000000000000000 ) ) ;
#15423=CIRCLE ( 'NONE', #4127, 5.000000000000000888 ) ;
#15430=CARTESIAN_POINT ( 'NONE',  ( -2.179449471770337432, -4.500000000000000000, -3.000000000000000000 ) ) ;
#15437=CARTESIAN_POINT ( 'NONE',  ( -2.816212223827430972, -7.500000000000002665, -15.81854889450412216 ) ) ;
#15455=DIRECTION ( 'NONE',  ( 0.000000000000000000, 0.000000000000000000, -1.000000000000000000 ) ) ;
#15461=CARTESIAN_POINT ( 'NONE',  ( -4.196046169205011722, 7.499999999999999112, -16.53685941778014978 ) ) ;
#15474=VECTOR ( 'NONE', #2599, 1000.000000000000000 ) ;
#15481=CARTESIAN_POINT ( 'NONE',  ( -6.500003738482100779, -7.499999999999348965, -12.10028435765593890 ) ) ;
#15488=EDGE_CURVE ( 'NONE', #18705, #13316, #9487, .T. ) ;
#15554=CARTESIAN_POINT ( 'NONE',  ( 6.538348415311013184, 7.500000000000000000, -12.00000000000000000 ) ) ;
#15559=DIRECTION ( 'NONE',  ( -1.000000000000000000, 0.000000000000000000, 0.000000000000000000 ) ) ;
#15585=LINE ( 'NONE', #4314, #4646 ) ;
#15615=FACE_OUTER_BOUND ( 'NONE', #6581, .T. ) ;
#15626=EDGE_LOOP ( 'NONE', ( #481, #10338, #1161, #13365, #14207, #9603 ) ) ;
#15637=CARTESIAN_POINT ( 'NONE',  ( 6.259160902251540648, 7.500000000000127898, -12.42139992667815562 ) ) ;
#15644=LINE ( 'NONE', #18801, #3293 ) ;
#15654=AXIS2_PLACEMENT_3D ( 'NONE', #8796, #7081, #14616 ) ;
#15669=( GEOMETRIC_REPRESENTATION_CONTEXT ( 3 ) GLOBAL_UNCERTAINTY_ASSIGNED_CONTEXT ( ( #8434 ) ) GLOBAL_UNIT_ASSIGNED_CONTEXT ( ( #2113, #18067, #3432 ) ) REPRESENTATION_CONTEXT ( 'NONE', 'WORKASPACE' ) );
#15704=ORIENTED_EDGE ( 'NONE', *, *, #4097, .T. ) ;
#15710=DIRECTION ( 'NONE',  ( 1.000000000000000000, 0.000000000000000000, 0.000000000000000000 ) ) ;
#15716=CARTESIAN_POINT ( 'NONE',  ( 0.000000000000000000, 0.000000000000000000, 0.000000000000000000 ) ) ;
#15724=ORIENTED_EDGE ( 'NONE', *, *, #11066, .T. ) ;
#15727=AXIS2_PLACEMENT_3D ( 'NONE', #15200, #6412, #10805 ) ;
#15737=CARTESIAN_POINT ( 'NONE',  ( 2.067729357296171688, 7.499999999999999112, -15.30380495029818988 ) ) ;
#15780=AXIS2_PLACEMENT_3D ( 'NONE', #11686, #10065, #11325 ) ;
#15821=ORIENTED_EDGE ( 'NONE', *, *, #11690, .F. ) ;
#15824=ORIENTED_EDGE ( 'NONE', *, *, #6731, .T. ) ;
#15827=ORIENTED_EDGE ( 'NONE', *, *, #17118, .T. ) ;
#15834=CARTESIAN_POINT ( 'NONE',  ( 3.606670283718163450, 7.499999999999999112, -16.27044756620607302 ) ) ;
#15836=CIRCLE ( 'NONE', #13440, 2.500000000000000000 ) ;
#15850=CARTESIAN_POINT ( 'NONE',  ( -20.00000000000000000, -2.500000000000000444, -16.99999999999999645 ) ) ;
#15889=CARTESIAN_POINT ( 'NONE',  ( 20.00000000000000000, 2.499999999999998668, -22.00000000000000000 ) ) ;
#15896=EDGE_CURVE ( 'NONE', #18879, #5818, #14851, .T. ) ;
#15910=DIRECTION ( 'NONE',  ( -1.000000000000000000, 0.000000000000000000, 0.000000000000000000 ) ) ;
#15922=DIRECTION ( 'NONE',  ( -1.000000000000000000, 6.938893903907228378E-16, 0.000000000000000000 ) ) ;
#15927=CARTESIAN_POINT ( 'NONE',  ( 5.856338620593967370, 7.500000000000129674, -12.72522090842645426 ) ) ;
#15931=EDGE_CURVE ( 'NONE', #4766, #322, #4891, .T. ) ;
#15967=CARTESIAN_POINT ( 'NONE',  ( 6.538348415311014072, -7.500000000000000888, -17.00000000000000000 ) ) ;
#15989=CIRCLE ( 'NONE', #10505, 5.000000000000000888 ) ;
#16031=SPHERICAL_SURFACE ( 'NONE', #528, 5.000000000000000000 ) ;
#16049=( GEOMETRIC_REPRESENTATION_CONTEXT ( 3 ) GLOBAL_UNCERTAINTY_ASSIGNED_CONTEXT ( ( #16266 ) ) GLOBAL_UNIT_ASSIGNED_CONTEXT ( ( #6264, #2155, #540 ) ) REPRESENTATION_CONTEXT ( 'NONE', 'WORKASPACE' ) );
#16054=FACE_OUTER_BOUND ( 'NONE', #15626, .T. ) ;
#16066=CARTESIAN_POINT ( 'NONE',  ( 2.117882332754172037, -7.500000000000000888, -15.34025089741903081 ) ) ;
#16071=VECTOR ( 'NONE', #12328, 1000.000000000000000 ) ;
#16089=ORIENTED_EDGE ( 'NONE', *, *, #17354, .F. ) ;
#16092=ORIENTED_EDGE ( 'NONE', *, *, #9862, .F. ) ;
#16150=CARTESIAN_POINT ( 'NONE',  ( -6.538348415311011408, 2.499999999999998224, -12.00000000000000000 ) ) ;
#16157=VECTOR ( 'NONE', #115, 1000.000000000000000 ) ;
#16166=CARTESIAN_POINT ( 'NONE',  ( 5.343731732830336867, -7.500000000000000888, -16.88485148858663365 ) ) ;
#16172=CARTESIAN_POINT ( 'NONE',  ( 0.000000000000000000, 2.499999999999998668, -22.00000000000000000 ) ) ;
#16184=EDGE_LOOP ( 'NONE', ( #9950, #770, #10963 ) ) ;
#16241=FACE_OUTER_BOUND ( 'NONE', #17285, .T. ) ;
#16246=CARTESIAN_POINT ( 'NONE',  ( -0.3448739086965367795, 7.500000000000000000, -14.22069309503974921 ) ) ;
#16248=CARTESIAN_POINT ( 'NONE',  ( -6.500524771654098366, 7.499999999999099387, -12.09892167832694199 ) ) ;
#16261=ORIENTED_EDGE ( 'NONE', *, *, #11124, .F. ) ;
#16266=UNCERTAINTY_MEASURE_WITH_UNIT (LENGTH_MEASURE( 1.000000000000000082E-05 ), #6264, 'distance_accuracy_value', 'NONE');
#16288=ORIENTED_EDGE ( 'NONE', *, *, #5563, .F. ) ;
#16307=CIRCLE ( 'NONE', #18725, 5.000000000000000000 ) ;
#16309=EDGE_CURVE ( 'NONE', #6378, #322, #13934, .T. ) ;
#16310=DIRECTION ( 'NONE',  ( 1.000000000000000000, 0.000000000000000000, 0.000000000000000000 ) ) ;
#16324=ORIENTED_EDGE ( 'NONE', *, *, #6731, .F. ) ;
#16332=CARTESIAN_POINT ( 'NONE',  ( 20.00000000000000000, -2.500000000000000444, -16.99999999999999645 ) ) ;
#16347=CARTESIAN_POINT ( 'NONE',  ( 1.823557580623806018, 7.500000000000000888, -15.12114310604040313 ) ) ;
#16348=DIRECTION ( 'NONE',  ( -0.000000000000000000, 1.000000000000000000, 0.000000000000000000 ) ) ;
#16367=CARTESIAN_POINT ( 'NONE',  ( 6.021941181548189803, -3.575661417670232822, -12.00000000127650246 ) ) ;
#16373=CARTESIAN_POINT ( 'NONE',  ( 0.000000000000000000, 0.000000000000000000, -13.00000000000000533 ) ) ;
#16446=CARTESIAN_POINT ( 'NONE',  ( -2.611515231136698034, 7.500000000000001776, -15.68397129924701794 ) ) ;
#16447=AXIS2_PLACEMENT_3D ( 'NONE', #2455, #6974, #15559 ) ;
#16458=VERTEX_POINT ( 'NONE', #15135 ) ;
#16464=CARTESIAN_POINT ( 'NONE',  ( -1.329112640582302607, -6.875529660588494352, -12.00000000371739084 ) ) ;
#16469=DIRECTION ( 'NONE',  ( -0.000000000000000000, -0.000000000000000000, 1.000000000000000000 ) ) ;
#16473=EDGE_CURVE ( 'NONE', #18879, #3494, #16844, .T. ) ;
#16531=VERTEX_POINT ( 'NONE', #15229 ) ;
#16544=CARTESIAN_POINT ( 'NONE',  ( -2.864513242452084274, 7.499999999999999112, -15.84899838955092655 ) ) ;
#16547=SURFACE_SIDE_STYLE ('',( #3628 ) ) ;
#16558=CARTESIAN_POINT ( 'NONE',  ( -4.482738663876439489, -5.389345431477982729, -11.99999999527192074 ) ) ;
#16584=DIRECTION ( 'NONE',  ( 0.000000000000000000, 0.000000000000000000, 1.000000000000000000 ) ) ;
#16629=CARTESIAN_POINT ( 'NONE',  ( -0.3286731010496698469, 6.995544057484794465, -12.00000000211882956 ) ) ;
#16642=CARTESIAN_POINT ( 'NONE',  ( 0.8060261380167486056, -7.499999999999904077, -13.05296413415621615 ) ) ;
#16648=CIRCLE ( 'NONE', #11759, 7.000000000000000000 ) ;
#16651=ADVANCED_FACE ( 'NONE', ( #14215 ), #6775, .F. ) ;
#16672=CARTESIAN_POINT ( 'NONE',  ( 0.000000000000000000, 0.000000000000000000, -12.00000000000000000 ) ) ;
#16696=CARTESIAN_POINT ( 'NONE',  ( -6.231098469233190329, -7.499999999999999112, -16.99999999999999645 ) ) ;
#16698=CARTESIAN_POINT ( 'NONE',  ( -20.00000000000000000, 2.499999999999998668, -17.00000000000000000 ) ) ;
#16706=VECTOR ( 'NONE', #18265, 1000.000000000000000 ) ;
#16711=VERTEX_POINT ( 'NONE', #2058 ) ;
#16725=CARTESIAN_POINT ( 'NONE',  ( -5.783659440658965423, 3.949482697158818389, -11.99999999872357748 ) ) ;
#16727=CONICAL_SURFACE ( 'NONE', #854, 2.500000000000000000, 1.029744258676656754 ) ;
#16729=FILL_AREA_STYLE ('',( #17978 ) ) ;
#16733=ORIENTED_EDGE ( 'NONE', *, *, #16473, .F. ) ;
#16740=CARTESIAN_POINT ( 'NONE',  ( -3.601232060343992014, -7.499999999999612754, -13.21583132166217744 ) ) ;
#16758=ADVANCED_FACE ( 'NONE', ( #13886 ), #5191, .T. ) ;
#16765=CIRCLE ( 'NONE', #7664, 5.000000000000000000 ) ;
#16777=VECTOR ( 'NONE', #12300, 1000.000000000000000 ) ;
#16788=CARTESIAN_POINT ( 'NONE',  ( 0.6293707761309761395, -7.500000000000001776, -14.32724244806440517 ) ) ;
#16789=ORIENTED_EDGE ( 'NONE', *, *, #4153, .F. ) ;
#16793=CARTESIAN_POINT ( 'NONE',  ( 20.00000000000000000, -2.500000000000000444, -22.00000000000000000 ) ) ;
#16801=ORIENTED_EDGE ( 'NONE', *, *, #1832, .F. ) ;
#16811=CARTESIAN_POINT ( 'NONE',  ( 0.03525595549292682984, 7.499999999999999112, -14.17755750872172271 ) ) ;
#16815=DIRECTION ( 'NONE',  ( 1.000000000000000000, 0.000000000000000000, -0.000000000000000000 ) ) ;
#16824=ORIENTED_EDGE ( 'NONE', *, *, #8028, .F. ) ;
#16826=CARTESIAN_POINT ( 'NONE',  ( -2.564349062531098067, -7.500000000000000888, -15.65236830614252028 ) ) ;
#16844=LINE ( 'NONE', #12353, #17012 ) ;
#16857=EDGE_CURVE ( 'NONE', #7506, #8066, #15836, .T. ) ;
#16869=ORIENTED_EDGE ( 'NONE', *, *, #9182, .T. ) ;
#16875=CARTESIAN_POINT ( 'NONE',  ( 0.1940040276537112751, -7.500000000000000000, -14.18536928022392019 ) ) ;
#16876=CARTESIAN_POINT ( 'NONE',  ( 25.00000000000000000, -7.500000000000000888, -16.99999999999999645 ) ) ;
#16880=EDGE_CURVE ( 'NONE', #1187, #9395, #16765, .T. ) ;
#16894=CARTESIAN_POINT ( 'NONE',  ( 20.00000000000000000, 2.499999999999998668, -16.99999999999999645 ) ) ;
#16899=DIRECTION ( 'NONE',  ( -1.000000000000000000, -0.000000000000000000, -6.938893903907227392E-16 ) ) ;
#16900=CARTESIAN_POINT ( 'NONE',  ( -0.6634400264848326900, 7.499999999999671374, -13.04619536630290533 ) ) ;
#16916=CARTESIAN_POINT ( 'NONE',  ( -4.449459268825699532, -7.500000000000000888, -16.63368482084344890 ) ) ;
#16945=ORIENTED_EDGE ( 'NONE', *, *, #5419, .F. ) ;
#16973=DIRECTION ( 'NONE',  ( 0.000000000000000000, 0.000000000000000000, -1.000000000000000000 ) ) ;
#16980=CIRCLE ( 'NONE', #5339, 5.000000000000000888 ) ;
#16998=CARTESIAN_POINT ( 'NONE',  ( 0.3372494957990315734, 7.499999999999999112, -14.22369192593357923 ) ) ;
#17002=CYLINDRICAL_SURFACE ( 'NONE', #15727, 5.000000000000000888 ) ;
#17012=VECTOR ( 'NONE', #7892, 1000.000000000000000 ) ;
#17020=CARTESIAN_POINT ( 'NONE',  ( -5.029793280284183155, -7.500000000000000888, -16.81208494724225133 ) ) ;
#17040=ORIENTED_EDGE ( 'NONE', *, *, #15246, .T. ) ;
#17060=DIRECTION ( 'NONE',  ( -1.000000000000000000, 0.000000000000000000, 0.000000000000000000 ) ) ;
#17087=CARTESIAN_POINT ( 'NONE',  ( 3.253466017773726904, 7.500000000000133227, -13.21345932477064622 ) ) ;
#17102=CARTESIAN_POINT ( 'NONE',  ( 0.000000000000000000, 0.000000000000000000, -3.000000000000000000 ) ) ;
#17106=CARTESIAN_POINT ( 'NONE',  ( -7.000000000000000000, 8.572527594031473190E-16, -12.00000000000000000 ) ) ;
#17118=EDGE_CURVE ( 'NONE', #8066, #7506, #6699, .T. ) ;
#17193=CARTESIAN_POINT ( 'NONE',  ( -6.499600586846986161, -2.601338725571163302, -12.00000000000000000 ) ) ;
#17218=EDGE_CURVE ( 'NONE', #4154, #1807, #10080, .T. ) ;
#17229=AXIS2_PLACEMENT_3D ( 'NONE', #18438, #3732, #2297 ) ;
#17247=DIRECTION ( 'NONE',  ( 0.000000000000000000, 0.000000000000000000, -1.000000000000000000 ) ) ;
#17249=DIRECTION ( 'NONE',  ( 1.000000000000000000, 0.000000000000000000, 0.000000000000000000 ) ) ;
#17265=CARTESIAN_POINT ( 'NONE',  ( 4.162578369387309074, 7.499999999999999112, -16.52352554129636886 ) ) ;
#17267=DIRECTION ( 'NONE',  ( 1.000000000000000000, -0.000000000000000000, -0.000000000000000000 ) ) ;
#17274=ORIENTED_EDGE ( 'NONE', *, *, #1832, .T. ) ;
#17285=EDGE_LOOP ( 'NONE', ( #18595, #1466, #13560, #8404 ) ) ;
#17314=CARTESIAN_POINT ( 'NONE',  ( 0.000000000000000000, 0.000000000000000000, -13.00000000000000533 ) ) ;
#17337=EDGE_CURVE ( 'NONE', #8559, #17372, #605, .T. ) ;
#17354=EDGE_CURVE ( 'NONE', #14283, #748, #2131, .T. ) ;
#17355=SPHERICAL_SURFACE ( 'NONE', #12655, 5.000000000000000000 ) ;
#17362=CARTESIAN_POINT ( 'NONE',  ( 0.4829358362135124927, 7.499999999999999112, -14.27056707468146435 ) ) ;
#17372=VERTEX_POINT ( 'NONE', #10514 ) ;
#17384=ORIENTED_EDGE ( 'NONE', *, *, #5419, .T. ) ;
#17395=DIRECTION ( 'NONE',  ( -0.000000000000000000, 0.000000000000000000, -1.000000000000000000 ) ) ;
#17403=CARTESIAN_POINT ( 'NONE',  ( 5.641944871949947427, -4.153144983956821079, -12.00000000256098254 ) ) ;
#17405=ORIENTED_EDGE ( 'NONE', *, *, #2048, .F. ) ;
#17408=ADVANCED_FACE ( 'NONE', ( #9172 ), #4389, .T. ) ;
#17409=ADVANCED_FACE ( 'NONE', ( #13181 ), #1923, .T. ) ;
#17502=FACE_OUTER_BOUND ( 'NONE', #14001, .T. ) ;
#17551=DIRECTION ( 'NONE',  ( -1.000000000000000000, 0.000000000000000000, 0.000000000000000000 ) ) ;
#17599=ORIENTED_EDGE ( 'NONE', *, *, #9512, .T. ) ;
#17619=AXIS2_PLACEMENT_3D ( 'NONE', #18117, #3679, #2161 ) ;
#17630=EDGE_CURVE ( 'NONE', #12766, #13344, #15171, .T. ) ;
#17649=VERTEX_POINT ( 'NONE', #2088 ) ;
#17653=DIRECTION ( 'NONE',  ( -6.938893903907228378E-16, -1.000000000000000000, 0.000000000000000000 ) ) ;
#17661=EDGE_CURVE ( 'NONE', #622, #5848, #8528, .T. ) ;
#17662=EDGE_CURVE ( 'NONE', #748, #14283, #16648, .T. ) ;
#17687=CARTESIAN_POINT ( 'NONE',  ( -5.934112841480000178, 7.499999999999999112, -16.97589560338757408 ) ) ;
#17703=ADVANCED_FACE ( 'NONE', ( #827 ), #12942, .F. ) ;
#17708=CARTESIAN_POINT ( 'NONE',  ( 4.576598828870276137, -7.499999999999999112, -13.14213029402371014 ) ) ;
#17762=CARTESIAN_POINT ( 'NONE',  ( -19.99999999999999645, 2.499999999999998668, -16.99999999999999645 ) ) ;
#17770=EDGE_LOOP ( 'NONE', ( #7170, #3316, #2758, #12299 ) ) ;
#17782=DIRECTION ( 'NONE',  ( -1.000000000000000000, 0.000000000000000000, 0.000000000000000000 ) ) ;
#17798=STYLED_ITEM ( 'NONE', ( #10998 ), #10500 ) ;
#17804=APPLICATION_CONTEXT ( 'automotive_design' ) ;
#17816=DIRECTION ( 'NONE',  ( -1.000000000000000000, 0.000000000000000000, 0.000000000000000000 ) ) ;
#17857=DIRECTION ( 'NONE',  ( -1.000000000000000000, 0.000000000000000000, 6.938893903907227392E-16 ) ) ;
#17876=CARTESIAN_POINT ( 'NONE',  ( 2.563381608035277370, 7.500000000000000000, -15.65171369207284435 ) ) ;
#17895=CARTESIAN_POINT ( 'NONE',  ( -2.826946895707799445, -6.438259034076553533, -12.00000001686866469 ) ) ;
#17975=CARTESIAN_POINT ( 'NONE',  ( 0.000000000000000000, 0.000000000000000000, -12.00000000000000000 ) ) ;
#17976=CARTESIAN_POINT ( 'NONE',  ( -5.308815406012119986, 7.500000000000000000, -12.96907596528355455 ) ) ;
#17978=FILL_AREA_STYLE_COLOUR ( '', #1641 ) ;
#17990=CARTESIAN_POINT ( 'NONE',  ( -1.089171355198575775, -7.500000000000000888, -14.58290923294939923 ) ) ;
#17999=DIRECTION ( 'NONE',  ( 1.734723475976806848E-16, 1.000000000000000000, -0.000000000000000000 ) ) ;
#18004=ORIENTED_EDGE ( 'NONE', *, *, #17662, .F. ) ;
#18012=ORIENTED_EDGE ( 'NONE', *, *, #2325, .F. ) ;
#18051=ORIENTED_EDGE ( 'NONE', *, *, #18671, .T. ) ;
#18061=CARTESIAN_POINT ( 'NONE',  ( 0.1112489676725757909, 7.500000000000000888, -14.17494330110304901 ) ) ;
#18063=CARTESIAN_POINT ( 'NONE',  ( -0.5390158121839171423, 6.982261029182147638, -11.99999999709518761 ) ) ;
#18067=( NAMED_UNIT ( * ) PLANE_ANGLE_UNIT ( ) SI_UNIT ( $, .RADIAN. ) );
#18081=CARTESIAN_POINT ( 'NONE',  ( 0.6292663627305138396, -7.500000000000000888, -14.32718894987486635 ) ) ;
#18101=EDGE_LOOP ( 'NONE', ( #13367, #7429, #11696, #16801 ) ) ;
#18117=CARTESIAN_POINT ( 'NONE',  ( -20.00000000000000000, -2.500000000000000444, -16.99999999999999645 ) ) ;
#18126=CARTESIAN_POINT ( 'NONE',  ( 4.478293880065215227, -7.500000000000001776, -16.64373187125687181 ) ) ;
#18136=VECTOR ( 'NONE', #1821, 1000.000000000000000 ) ;
#18153=CARTESIAN_POINT ( 'NONE',  ( -0.6292663627301623430, 7.499999999999999112, -14.32718894987469938 ) ) ;
#18171=CARTESIAN_POINT ( 'NONE',  ( -0.7597029211758296041, -7.500000000000000888, -14.39758526244282599 ) ) ;
#18178=DIRECTION ( 'NONE',  ( 0.000000000000000000, -1.000000000000000000, 0.000000000000000000 ) ) ;
#18195=EDGE_CURVE ( 'NONE', #8066, #5247, #8415, .T. ) ;
#18201=SHAPE_DEFINITION_REPRESENTATION ( #13324, #11674 ) ;
#18202=FILL_AREA_STYLE ('',( #3382 ) ) ;
#18219=CARTESIAN_POINT ( 'NONE',  ( -5.322906077793310153, -7.500000000000001776, -16.88078391064166439 ) ) ;
#18229=DIRECTION ( 'NONE',  ( 0.000000000000000000, -1.000000000000000000, 0.000000000000000000 ) ) ;
#18249=CARTESIAN_POINT ( 'NONE',  ( -2.576507258268692535, 7.499999999999999112, -13.18245040793292233 ) ) ;
#18262=CARTESIAN_POINT ( 'NONE',  ( -5.275788075193909243, -7.500000000000000888, -12.98022329939712094 ) ) ;
#18265=DIRECTION ( 'NONE',  ( 1.000000000000000000, -0.000000000000000000, -0.000000000000000000 ) ) ;
#18293=CARTESIAN_POINT ( 'NONE',  ( 25.00000000000000000, -7.500000000000000888, -17.00000000000000000 ) ) ;
#18309=CARTESIAN_POINT ( 'NONE',  ( -1.333872087798559480, -7.500000000000001776, -14.76174338479138726 ) ) ;
#18332=CARTESIAN_POINT ( 'NONE',  ( -2.953963787679199537, 6.378445150919402451, -12.00000001548991158 ) ) ;
#18354=CARTESIAN_POINT ( 'NONE',  ( 0.000000000000000000, 0.000000000000000000, -13.00000000000000533 ) ) ;
#18419=CARTESIAN_POINT ( 'NONE',  ( 1.329112640582405191, 6.875529660588472147, -12.00000000371739439 ) ) ;
#18427=ORIENTED_EDGE ( 'NONE', *, *, #17630, .F. ) ;
#18438=CARTESIAN_POINT ( 'NONE',  ( 25.00000000000000000, 2.499999999999998668, -17.00000000000000000 ) ) ;
#18487=CARTESIAN_POINT ( 'NONE',  ( 0.000000000000000000, 0.000000000000000000, -12.00000000000000000 ) ) ;
#18490=ADVANCED_FACE ( 'NONE', ( #2111 ), #17002, .T. ) ;
#18513=VECTOR ( 'NONE', #10625, 1000.000000000000000 ) ;
#18515=CARTESIAN_POINT ( 'NONE',  ( 4.238775304281403145, 7.500000000000264677, -13.18441022661325945 ) ) ;
#18535=CARTESIAN_POINT ( 'NONE',  ( -6.538348415310989203, -7.500000000000000000, -12.00000000000006040 ) ) ;
#18571=DIRECTION ( 'NONE',  ( 0.000000000000000000, 1.000000000000000000, 0.000000000000000000 ) ) ;
#18595=ORIENTED_EDGE ( 'NONE', *, *, #11066, .F. ) ;
#18596=DIRECTION ( 'NONE',  ( -0.000000000000000000, 0.000000000000000000, 1.000000000000000000 ) ) ;
#18604=CARTESIAN_POINT ( 'NONE',  ( 5.275788075193746707, 7.499999999999999112, -12.98022329939734298 ) ) ;
#18625=DIRECTION ( 'NONE',  ( -1.000000000000000000, 0.000000000000000000, 0.000000000000000000 ) ) ;
#18671=EDGE_CURVE ( 'NONE', #9678, #5818, #5598, .T. ) ;
#18694=CARTESIAN_POINT ( 'NONE',  ( 5.031681560115344176, 4.880796135282181147, -12.00000000472804196 ) ) ;
#18705=VERTEX_POINT ( 'NONE', #270 ) ;
#18717=DIRECTION ( 'NONE',  ( 0.000000000000000000, 0.000000000000000000, -1.000000000000000000 ) ) ;
#18725=AXIS2_PLACEMENT_3D ( 'NONE', #12803, #18717, #18625 ) ;
#18780=VERTEX_POINT ( 'NONE', #16793 ) ;
#18793=CARTESIAN_POINT ( 'NONE',  ( 6.144877202870933530, 7.499999999999866773, -12.52666336607983233 ) ) ;
#18801=CARTESIAN_POINT ( 'NONE',  ( -7.000000000000000000, 8.572527594031473190E-16, -12.00000000000000000 ) ) ;
#18832=EDGE_CURVE ( 'NONE', #5818, #4766, #6388, .T. ) ;
#18879=VERTEX_POINT ( 'NONE', #15175 ) ;
#18897=VERTEX_POINT ( 'NONE', #8464 ) ;
ENDSEC;
END-ISO-10303-21;
